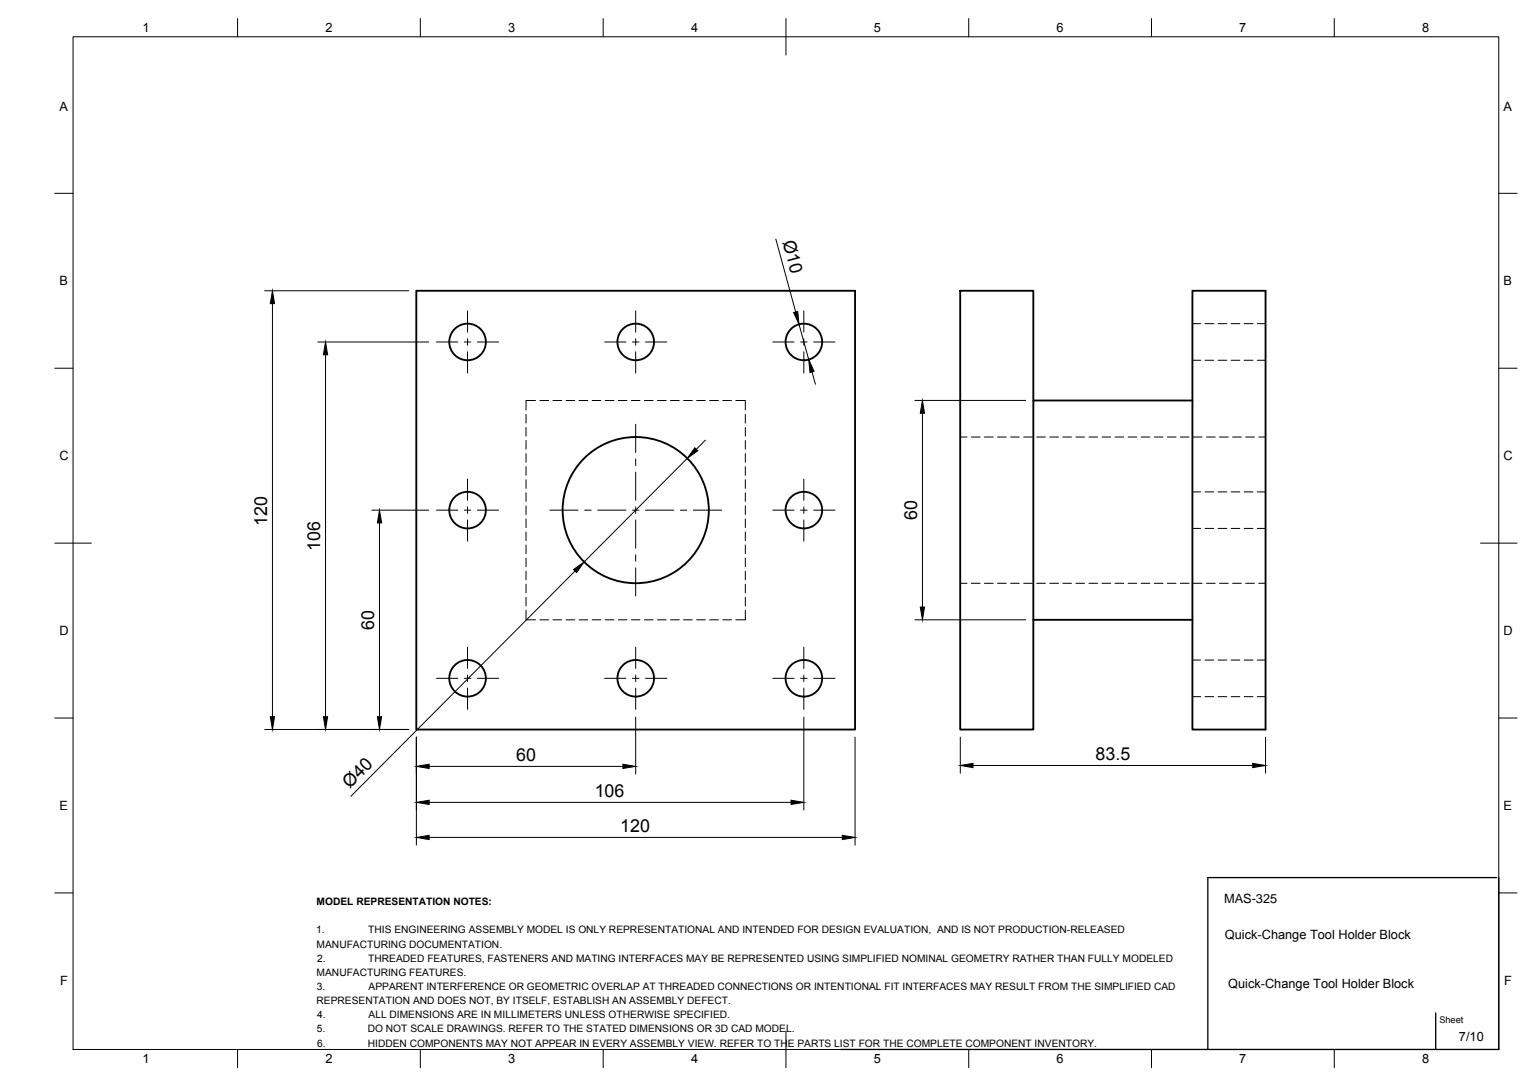
ISO-10303-21;
HEADER;
FILE_DESCRIPTION (('STEP AP214'),
    '1' );
FILE_NAME ('Quick-Change Tool Holder Block.step',
    '2026-10-08T01:23:29',
    ( '' ),
    ( '' ),
    'SwSTEP 2.0',
    'SolidWorks 2025',
    '' );
FILE_SCHEMA (( 'AUTOMOTIVE_DESIGN' ));
ENDSEC;

DATA;
#8=DIRECTION ( 'NONE',  ( 0.000000000000000000, 0.000000000000000000, -1.000000000000000000 ) ) ;
#231=DIRECTION ( 'NONE',  ( -0.000000000000000000, 1.000000000000000000, -0.000000000000000000 ) ) ;
#235=AXIS2_PLACEMENT_3D ( 'NONE', #29797, #45849, #41895 ) ;
#469=EDGE_LOOP ( 'NONE', ( #38599, #878, #20633, #16037 ) ) ;
#500=AXIS2_PLACEMENT_3D ( 'NONE', #889, #41099, #37682 ) ;
#509=DIRECTION ( 'NONE',  ( 0.000000000000000000, 1.000000000000000000, 0.000000000000000000 ) ) ;
#511=DIRECTION ( 'NONE',  ( 1.000000000000000000, -0.000000000000000000, 0.000000000000000000 ) ) ;
#519=CIRCLE ( 'NONE', #6403, 4.999999999999997335 ) ;
#529=( GEOMETRIC_REPRESENTATION_CONTEXT ( 3 ) GLOBAL_UNCERTAINTY_ASSIGNED_CONTEXT ( ( #31631 ) ) GLOBAL_UNIT_ASSIGNED_CONTEXT ( ( #33419, #33134, #45500 ) ) REPRESENTATION_CONTEXT ( 'NONE', 'WORKASPACE' ) );
#610=ADVANCED_FACE ( 'NONE', ( #10402 ), #26946, .F. ) ;
#630=ORIENTED_EDGE ( 'NONE', *, *, #47620, .F. ) ;
#643=ORIENTED_EDGE ( 'NONE', *, *, #44701, .T. ) ;
#683=EDGE_LOOP ( 'NONE', ( #15147, #11656, #13583, #27814 ) ) ;
#690=FACE_OUTER_BOUND ( 'NONE', #23025, .T. ) ;
#746=CARTESIAN_POINT ( 'NONE',  ( -46.00000000000000711, 0.000000000000000000, 8.673617379884035472E-15 ) ) ;
#755=VERTEX_POINT ( 'NONE', #51930 ) ;
#805=CARTESIAN_POINT ( 'NONE',  ( 46.00000000000000711, 0.000000000000000000, 41.00000000000000000 ) ) ;
#835=DIRECTION ( 'NONE',  ( 0.000000000000000000, 1.000000000000000000, 0.000000000000000000 ) ) ;
#848=ORIENTED_EDGE ( 'NONE', *, *, #2477, .T. ) ;
#878=ORIENTED_EDGE ( 'NONE', *, *, #33812, .F. ) ;
#889=CARTESIAN_POINT ( 'NONE',  ( 46.00000000000000711, 20.00000000000000000, 46.00000000000000000 ) ) ;
#902=EDGE_CURVE ( 'NONE', #32022, #7418, #51728, .T. ) ;
#905=DIRECTION ( 'NONE',  ( 0.000000000000000000, 0.000000000000000000, 1.000000000000000000 ) ) ;
#956=DIRECTION ( 'NONE',  ( 0.000000000000000000, 0.000000000000000000, -1.000000000000000000 ) ) ;
#984=CARTESIAN_POINT ( 'NONE',  ( -46.00000000000000711, 20.00000000000000000, 51.00000000000000000 ) ) ;
#1030=CIRCLE ( 'NONE', #8567, 4.999999999999997335 ) ;
#1039=EDGE_LOOP ( 'NONE', ( #32156, #50027, #34356, #41255 ) ) ;
#1073=SURFACE_SIDE_STYLE ('',( #5041 ) ) ;
#1080=PLANE ( 'NONE',  #27310 ) ;
#1090=DIRECTION ( 'NONE',  ( 0.000000000000000000, 0.000000000000000000, 1.000000000000000000 ) ) ;
#1094=DIRECTION ( 'NONE',  ( 0.000000000000000000, 0.000000000000000000, 1.000000000000000000 ) ) ;
#1126=VERTEX_POINT ( 'NONE', #22089 ) ;
#1141=MANIFOLD_SOLID_BREP ( 'Cut-Extrude1', #17058 ) ;
#1185=EDGE_LOOP ( 'NONE', ( #30507, #5255 ) ) ;
#1316=LINE ( 'NONE', #8951, #2361 ) ;
#1322=ORIENTED_EDGE ( 'NONE', *, *, #37609, .F. ) ;
#1346=CARTESIAN_POINT ( 'NONE',  ( -60.00000000000000000, 20.00000000000000000, 60.00000000000000711 ) ) ;
#1349=VERTEX_POINT ( 'NONE', #40428 ) ;
#1372=STYLED_ITEM ( 'NONE', ( #29978 ), #1141 ) ;
#1532=DIRECTION ( 'NONE',  ( 0.000000000000000000, -1.000000000000000000, 0.000000000000000000 ) ) ;
#1533=DIRECTION ( 'NONE',  ( 0.000000000000000000, 0.000000000000000000, -1.000000000000000000 ) ) ;
#1580=CARTESIAN_POINT ( 'NONE',  ( -60.00000000000000000, 0.000000000000000000, 60.00000000000000711 ) ) ;
#1620=DIRECTION ( 'NONE',  ( 1.000000000000000000, -0.000000000000000000, 0.000000000000000000 ) ) ;
#1628=LINE ( 'NONE', #13193, #27463 ) ;
#1634=ORIENTED_EDGE ( 'NONE', *, *, #11718, .F. ) ;
#1637=EDGE_CURVE ( 'NONE', #4347, #48702, #44495, .T. ) ;
#1686=ORIENTED_EDGE ( 'NONE', *, *, #8609, .T. ) ;
#1690=FACE_OUTER_BOUND ( 'NONE', #43640, .T. ) ;
#1791=DIRECTION ( 'NONE',  ( 0.000000000000000000, 0.000000000000000000, 1.000000000000000000 ) ) ;
#1796=DIRECTION ( 'NONE',  ( 0.000000000000000000, 0.000000000000000000, -1.000000000000000000 ) ) ;
#1921=EDGE_CURVE ( 'NONE', #24400, #35572, #31639, .T. ) ;
#1968=CARTESIAN_POINT ( 'NONE',  ( 46.00000000000000000, 20.00000000000000000, -4.999999999999997335 ) ) ;
#2088=VERTEX_POINT ( 'NONE', #36530 ) ;
#2096=DIRECTION ( 'NONE',  ( 0.000000000000000000, -1.000000000000000000, 0.000000000000000000 ) ) ;
#2101=VERTEX_POINT ( 'NONE', #805 ) ;
#2131=DIRECTION ( 'NONE',  ( 0.000000000000000000, 1.000000000000000000, 0.000000000000000000 ) ) ;
#2170=DIRECTION ( 'NONE',  ( 1.000000000000000000, -0.000000000000000000, 0.000000000000000000 ) ) ;
#2214=DIRECTION ( 'NONE',  ( 0.000000000000000000, 1.000000000000000000, 0.000000000000000000 ) ) ;
#2313=AXIS2_PLACEMENT_3D ( 'NONE', #18632, #34644, #50691 ) ;
#2361=VECTOR ( 'NONE', #24717, 1000.000000000000000 ) ;
#2426=CARTESIAN_POINT ( 'NONE',  ( 46.00000000000000000, 20.00000000000000000, 0.000000000000000000 ) ) ;
#2477=EDGE_CURVE ( 'NONE', #17289, #7125, #26422, .T. ) ;
#2494=CIRCLE ( 'NONE', #9212, 4.999999999999997335 ) ;
#2589=CARTESIAN_POINT ( 'NONE',  ( 0.000000000000000000, 0.000000000000000000, 0.000000000000000000 ) ) ;
#2614=ORIENTED_EDGE ( 'NONE', *, *, #31482, .F. ) ;
#2675=VECTOR ( 'NONE', #3987, 1000.000000000000000 ) ;
#2678=CARTESIAN_POINT ( 'NONE',  ( -46.00000000000000711, 0.000000000000000000, 51.00000000000000000 ) ) ;
#2740=UNCERTAINTY_MEASURE_WITH_UNIT (LENGTH_MEASURE( 1.000000000000000082E-05 ), #29982, 'distance_accuracy_value', 'NONE');
#2781=FACE_BOUND ( 'NONE', #44782, .T. ) ;
#2946=AXIS2_PLACEMENT_3D ( 'NONE', #746, #12029, #48846 ) ;
#2982=EDGE_LOOP ( 'NONE', ( #34516, #40352, #15843, #39033 ) ) ;
#2988=VECTOR ( 'NONE', #2170, 1000.000000000000000 ) ;
#3042=FACE_BOUND ( 'NONE', #22300, .T. ) ;
#3127=ORIENTED_EDGE ( 'NONE', *, *, #18949, .T. ) ;
#3185=FACE_OUTER_BOUND ( 'NONE', #37672, .T. ) ;
#3397=DIRECTION ( 'NONE',  ( 0.000000000000000000, 1.000000000000000000, 0.000000000000000000 ) ) ;
#3409=EDGE_CURVE ( 'NONE', #44223, #31469, #13220, .T. ) ;
#3423=DIRECTION ( 'NONE',  ( 0.000000000000000000, 0.000000000000000000, 1.000000000000000000 ) ) ;
#3531=CARTESIAN_POINT ( 'NONE',  ( 3.686287386450715076E-15, 20.00000000000000000, -51.00000000000000711 ) ) ;
#3541=CARTESIAN_POINT ( 'NONE',  ( -46.00000000000000711, 20.00000000000000000, 46.00000000000000000 ) ) ;
#3568=ORIENTED_EDGE ( 'NONE', *, *, #4402, .F. ) ;
#3630=CARTESIAN_POINT ( 'NONE',  ( 60.00000000000001421, -43.50000000000000000, 0.000000000000000000 ) ) ;
#3641=ORIENTED_EDGE ( 'NONE', *, *, #27551, .T. ) ;
#3670=DIRECTION ( 'NONE',  ( -0.000000000000000000, -1.000000000000000000, -0.000000000000000000 ) ) ;
#3714=CARTESIAN_POINT ( 'NONE',  ( 0.000000000000000000, 0.000000000000000000, 0.000000000000000000 ) ) ;
#3813=AXIS2_PLACEMENT_3D ( 'NONE', #22588, #41779, #50196 ) ;
#3855=DIRECTION ( 'NONE',  ( 0.000000000000000000, 0.000000000000000000, -1.000000000000000000 ) ) ;
#3861=ORIENTED_EDGE ( 'NONE', *, *, #27551, .F. ) ;
#3882=VECTOR ( 'NONE', #3670, 1000.000000000000000 ) ;
#3883=CYLINDRICAL_SURFACE ( 'NONE', #28633, 4.999999999999997335 ) ;
#3895=VECTOR ( 'NONE', #11796, 1000.000000000000000 ) ;
#3902=ORIENTED_EDGE ( 'NONE', *, *, #34227, .F. ) ;
#3904=LINE ( 'NONE', #3630, #38504 ) ;
#3936=CARTESIAN_POINT ( 'NONE',  ( 0.000000000000000000, -63.50000000000000000, 0.000000000000000000 ) ) ;
#3954=CIRCLE ( 'NONE', #45083, 4.999999999999997335 ) ;
#3985=CARTESIAN_POINT ( 'NONE',  ( -60.00000000000000000, 20.00000000000000000, -60.00000000000000711 ) ) ;
#3987=DIRECTION ( 'NONE',  ( -0.000000000000000000, -1.000000000000000000, -0.000000000000000000 ) ) ;
#4040=VECTOR ( 'NONE', #41244, 1000.000000000000000 ) ;
#4073=FACE_OUTER_BOUND ( 'NONE', #29955, .T. ) ;
#4079=ORIENTED_EDGE ( 'NONE', *, *, #24879, .T. ) ;
#4080=CARTESIAN_POINT ( 'NONE',  ( 46.00000000000000711, 0.000000000000000000, -41.00000000000000000 ) ) ;
#4147=EDGE_CURVE ( 'NONE', #15921, #22734, #9361, .T. ) ;
#4244=LINE ( 'NONE', #7662, #2675 ) ;
#4347=VERTEX_POINT ( 'NONE', #31648 ) ;
#4402=EDGE_CURVE ( 'NONE', #12957, #38011, #44515, .T. ) ;
#4405=DIRECTION ( 'NONE',  ( -0.000000000000000000, -1.000000000000000000, -0.000000000000000000 ) ) ;
#4414=EDGE_CURVE ( 'NONE', #28503, #18767, #48724, .T. ) ;
#4431=ORIENTED_EDGE ( 'NONE', *, *, #23553, .F. ) ;
#4572=CARTESIAN_POINT ( 'NONE',  ( 60.00000000000001421, 0.000000000000000000, 60.00000000000000711 ) ) ;
#4693=FACE_BOUND ( 'NONE', #20510, .T. ) ;
#4770=ORIENTED_EDGE ( 'NONE', *, *, #41010, .T. ) ;
#4804=ORIENTED_EDGE ( 'NONE', *, *, #25842, .T. ) ;
#4819=EDGE_CURVE ( 'NONE', #1349, #12957, #519, .T. ) ;
#4931=EDGE_LOOP ( 'NONE', ( #26759, #38319, #25353, #4431 ) ) ;
#4984=PRODUCT_CONTEXT ( 'NONE', #41108, 'mechanical' ) ;
#5041=SURFACE_STYLE_FILL_AREA ( #49956 ) ;
#5146=VERTEX_POINT ( 'NONE', #20149 ) ;
#5255=ORIENTED_EDGE ( 'NONE', *, *, #7025, .T. ) ;
#5265=CARTESIAN_POINT ( 'NONE',  ( 3.686287386450715076E-15, 0.000000000000000000, -51.00000000000000711 ) ) ;
#5492=VERTEX_POINT ( 'NONE', #38955 ) ;
#5593=ORIENTED_EDGE ( 'NONE', *, *, #21466, .F. ) ;
#5636=DIRECTION ( 'NONE',  ( 0.000000000000000000, 0.000000000000000000, -1.000000000000000000 ) ) ;
#5643=CIRCLE ( 'NONE', #22389, 4.999999999999997335 ) ;
#5650=CYLINDRICAL_SURFACE ( 'NONE', #44597, 4.999999999999997335 ) ;
#5685=CARTESIAN_POINT ( 'NONE',  ( 46.00000000000000711, 20.00000000000000000, -41.00000000000000000 ) ) ;
#5691=EDGE_LOOP ( 'NONE', ( #30462, #46109 ) ) ;
#5693=ORIENTED_EDGE ( 'NONE', *, *, #44701, .F. ) ;
#5706=DIRECTION ( 'NONE',  ( 0.000000000000000000, 0.000000000000000000, -1.000000000000000000 ) ) ;
#5754=EDGE_CURVE ( 'NONE', #12927, #38011, #3954, .T. ) ;
#5761=CARTESIAN_POINT ( 'NONE',  ( 46.00000000000000711, 0.000000000000000000, 46.00000000000000000 ) ) ;
#5767=DIRECTION ( 'NONE',  ( 0.000000000000000000, 1.000000000000000000, 0.000000000000000000 ) ) ;
#5781=VECTOR ( 'NONE', #38082, 1000.000000000000000 ) ;
#5784=FACE_BOUND ( 'NONE', #7278, .T. ) ;
#5789=EDGE_CURVE ( 'NONE', #7450, #24959, #1628, .T. ) ;
#5792=DIRECTION ( 'NONE',  ( 0.000000000000000000, 0.000000000000000000, 1.000000000000000000 ) ) ;
#5818=CARTESIAN_POINT ( 'NONE',  ( 46.00000000000000000, 0.000000000000000000, 4.999999999999997335 ) ) ;
#5827=CARTESIAN_POINT ( 'NONE',  ( -60.00000000000000000, 20.00000000000000000, 60.00000000000000711 ) ) ;
#5888=PRODUCT ( 'Quick-Change Tool Holder Block', 'Quick-Change Tool Holder Block', '', ( #4984 ) ) ;
#5895=ORIENTED_EDGE ( 'NONE', *, *, #17945, .T. ) ;
#5901=AXIS2_PLACEMENT_3D ( 'NONE', #21940, #30584, #50842 ) ;
#6015=DIRECTION ( 'NONE',  ( 0.000000000000000000, -1.000000000000000000, 0.000000000000000000 ) ) ;
#6058=CARTESIAN_POINT ( 'NONE',  ( 0.000000000000000000, -43.50000000000000000, 60.00000000000000711 ) ) ;
#6066=CARTESIAN_POINT ( 'NONE',  ( -46.00000000000000711, 20.00000000000000000, 51.00000000000000000 ) ) ;
#6079=AXIS2_PLACEMENT_3D ( 'NONE', #11818, #39421, #3423 ) ;
#6101=EDGE_CURVE ( 'NONE', #39324, #2101, #27838, .T. ) ;
#6133=CARTESIAN_POINT ( 'NONE',  ( 0.000000000000000000, -63.50000000000000000, 60.00000000000000711 ) ) ;
#6145=VERTEX_POINT ( 'NONE', #39918 ) ;
#6217=CARTESIAN_POINT ( 'NONE',  ( 60.00000000000001421, 20.00000000000000000, 60.00000000000000711 ) ) ;
#6247=ORIENTED_EDGE ( 'NONE', *, *, #1637, .T. ) ;
#6348=AXIS2_PLACEMENT_3D ( 'NONE', #34789, #46647, #41718 ) ;
#6392=CARTESIAN_POINT ( 'NONE',  ( -46.00000000000000711, 20.00000000000000000, 41.00000000000000000 ) ) ;
#6403=AXIS2_PLACEMENT_3D ( 'NONE', #26477, #37548, #1791 ) ;
#6461=AXIS2_PLACEMENT_3D ( 'NONE', #41940, #49327, #37993 ) ;
#6502=ORIENTED_EDGE ( 'NONE', *, *, #34896, .F. ) ;
#6529=DIRECTION ( 'NONE',  ( 0.000000000000000000, 1.000000000000000000, -0.000000000000000000 ) ) ;
#6548=ORIENTED_EDGE ( 'NONE', *, *, #40003, .F. ) ;
#6553=CARTESIAN_POINT ( 'NONE',  ( -46.00000000000000711, 0.000000000000000000, 46.00000000000000000 ) ) ;
#6561=FACE_OUTER_BOUND ( 'NONE', #21554, .T. ) ;
#6707=ORIENTED_EDGE ( 'NONE', *, *, #7167, .T. ) ;
#6734=EDGE_CURVE ( 'NONE', #5146, #10970, #33743, .T. ) ;
#6854=EDGE_CURVE ( 'NONE', #51787, #22734, #42666, .T. ) ;
#7025=EDGE_CURVE ( 'NONE', #7418, #32022, #49672, .T. ) ;
#7068=CARTESIAN_POINT ( 'NONE',  ( 46.00000000000000711, 0.000000000000000000, -46.00000000000000000 ) ) ;
#7093=CARTESIAN_POINT ( 'NONE',  ( 3.686287386450715076E-15, 20.00000000000000000, -46.00000000000000711 ) ) ;
#7111=VECTOR ( 'NONE', #5767, 1000.000000000000000 ) ;
#7125=VERTEX_POINT ( 'NONE', #46052 ) ;
#7126=EDGE_LOOP ( 'NONE', ( #30101, #33075, #43603, #25151 ) ) ;
#7149=ORIENTED_EDGE ( 'NONE', *, *, #48869, .T. ) ;
#7161=CIRCLE ( 'NONE', #27287, 4.999999999999997335 ) ;
#7167=EDGE_CURVE ( 'NONE', #32303, #51023, #36261, .T. ) ;
#7209=CARTESIAN_POINT ( 'NONE',  ( 60.00000000000001421, -63.50000000000000000, 60.00000000000000711 ) ) ;
#7264=DIRECTION ( 'NONE',  ( -0.000000000000000000, -1.000000000000000000, -0.000000000000000000 ) ) ;
#7278=EDGE_LOOP ( 'NONE', ( #48814, #44338 ) ) ;
#7334=ADVANCED_FACE ( 'NONE', ( #32309 ), #40203, .F. ) ;
#7418=VERTEX_POINT ( 'NONE', #37037 ) ;
#7450=VERTEX_POINT ( 'NONE', #13913 ) ;
#7488=VECTOR ( 'NONE', #38142, 1000.000000000000000 ) ;
#7497=CYLINDRICAL_SURFACE ( 'NONE', #35759, 4.999999999999997335 ) ;
#7503=LINE ( 'NONE', #8008, #28662 ) ;
#7516=FACE_BOUND ( 'NONE', #18343, .T. ) ;
#7524=ORIENTED_EDGE ( 'NONE', *, *, #44163, .F. ) ;
#7547=ORIENTED_EDGE ( 'NONE', *, *, #36563, .F. ) ;
#7557=ORIENTED_EDGE ( 'NONE', *, *, #37236, .T. ) ;
#7662=CARTESIAN_POINT ( 'NONE',  ( 46.00000000000000000, 20.00000000000000000, 4.999999999999997335 ) ) ;
#7765=PLANE ( 'NONE',  #14213 ) ;
#8008=CARTESIAN_POINT ( 'NONE',  ( 0.000000000000000000, -43.50000000000000000, 30.00000000000000355 ) ) ;
#8064=DIRECTION ( 'NONE',  ( 0.000000000000000000, 0.000000000000000000, -1.000000000000000000 ) ) ;
#8088=MECHANICAL_DESIGN_GEOMETRIC_PRESENTATION_REPRESENTATION('',(#1372),#529);
#8215=CARTESIAN_POINT ( 'NONE',  ( -60.00000000000000000, -63.50000000000000000, 60.00000000000000711 ) ) ;
#8284=AXIS2_PLACEMENT_3D ( 'NONE', #30164, #30408, #1533 ) ;
#8332=CYLINDRICAL_SURFACE ( 'NONE', #28030, 4.999999999999997335 ) ;
#8342=AXIS2_PLACEMENT_3D ( 'NONE', #33031, #17022, #40378 ) ;
#8393=CARTESIAN_POINT ( 'NONE',  ( -60.00000000000000000, 20.00000000000000000, 60.00000000000000711 ) ) ;
#8412=EDGE_LOOP ( 'NONE', ( #41893, #848 ) ) ;
#8438=DIRECTION ( 'NONE',  ( 1.000000000000000000, 0.000000000000000000, 0.000000000000000000 ) ) ;
#8551=EDGE_CURVE ( 'NONE', #23514, #28503, #43677, .T. ) ;
#8567=AXIS2_PLACEMENT_3D ( 'NONE', #48358, #509, #40450 ) ;
#8609=EDGE_CURVE ( 'NONE', #2088, #36416, #37552, .T. ) ;
#8665=CARTESIAN_POINT ( 'NONE',  ( 1.734723475976807094E-15, 20.00000000000000000, 41.00000000000000711 ) ) ;
#8716=FACE_BOUND ( 'NONE', #1185, .T. ) ;
#8752=PRODUCT_DEFINITION ( 'UNKNOWN', '', #25890, #46912 ) ;
#8951=CARTESIAN_POINT ( 'NONE',  ( -30.00000000000000000, -43.50000000000000000, 30.00000000000000355 ) ) ;
#8988=PLANE ( 'NONE',  #17210 ) ;
#9019=AXIS2_PLACEMENT_3D ( 'NONE', #30402, #43540, #46452 ) ;
#9124=EDGE_CURVE ( 'NONE', #35572, #24400, #23996, .T. ) ;
#9162=CARTESIAN_POINT ( 'NONE',  ( -46.00000000000000711, 20.00000000000000000, -46.00000000000000000 ) ) ;
#9166=DIRECTION ( 'NONE',  ( 0.000000000000000000, 0.000000000000000000, -1.000000000000000000 ) ) ;
#9212=AXIS2_PLACEMENT_3D ( 'NONE', #2426, #30523, #22394 ) ;
#9268=EDGE_LOOP ( 'NONE', ( #38964, #27022 ) ) ;
#9361=LINE ( 'NONE', #41927, #24178 ) ;
#9407=CIRCLE ( 'NONE', #36251, 4.999999999999997335 ) ;
#9439=CARTESIAN_POINT ( 'NONE',  ( 4.298610786024391605E-15, 20.00000000000000000, -41.00000000000000711 ) ) ;
#9671=AXIS2_PLACEMENT_3D ( 'NONE', #40075, #48759, #36662 ) ;
#9712=VECTOR ( 'NONE', #27639, 1000.000000000000000 ) ;
#9733=ORIENTED_EDGE ( 'NONE', *, *, #7167, .F. ) ;
#9982=DIRECTION ( 'NONE',  ( 0.000000000000000000, 1.000000000000000000, 0.000000000000000000 ) ) ;
#10076=ORIENTED_EDGE ( 'NONE', *, *, #21894, .T. ) ;
#10114=CARTESIAN_POINT ( 'NONE',  ( 30.00000000000000711, 0.000000000000000000, -30.00000000000000355 ) ) ;
#10243=AXIS2_PLACEMENT_3D ( 'NONE', #46644, #46908, #22717 ) ;
#10276=LINE ( 'NONE', #34446, #28627 ) ;
#10402=FACE_OUTER_BOUND ( 'NONE', #33728, .T. ) ;
#10425=ADVANCED_FACE ( 'NONE', ( #48600 ), #24662, .F. ) ;
#10445=DIRECTION ( 'NONE',  ( 0.000000000000000000, 0.000000000000000000, -1.000000000000000000 ) ) ;
#10511=AXIS2_PLACEMENT_3D ( 'NONE', #9162, #44633, #25189 ) ;
#10565=DIRECTION ( 'NONE',  ( -0.000000000000000000, -1.000000000000000000, -0.000000000000000000 ) ) ;
#10748=CARTESIAN_POINT ( 'NONE',  ( -60.00000000000000000, 20.00000000000000000, 60.00000000000000711 ) ) ;
#10832=EDGE_CURVE ( 'NONE', #6145, #23787, #1316, .T. ) ;
#10852=CIRCLE ( 'NONE', #8342, 4.999999999999997335 ) ;
#10928=DIRECTION ( 'NONE',  ( 0.000000000000000000, 0.000000000000000000, 1.000000000000000000 ) ) ;
#10970=VERTEX_POINT ( 'NONE', #47805 ) ;
#11051=VECTOR ( 'NONE', #33995, 1000.000000000000000 ) ;
#11070=CARTESIAN_POINT ( 'NONE',  ( 2.347046875550483230E-15, 20.00000000000000000, 51.00000000000000711 ) ) ;
#11100=CARTESIAN_POINT ( 'NONE',  ( -60.00000000000000000, 0.000000000000000000, 60.00000000000000711 ) ) ;
#11107=PLANE ( 'NONE',  #19321 ) ;
#11209=CARTESIAN_POINT ( 'NONE',  ( -46.00000000000000711, 0.000000000000000000, 41.00000000000000000 ) ) ;
#11223=EDGE_CURVE ( 'NONE', #33816, #30271, #34168, .T. ) ;
#11297=DIRECTION ( 'NONE',  ( -0.000000000000000000, -1.000000000000000000, -0.000000000000000000 ) ) ;
#11322=CIRCLE ( 'NONE', #10511, 4.999999999999997335 ) ;
#11435=DIRECTION ( 'NONE',  ( 0.000000000000000000, -1.000000000000000000, 0.000000000000000000 ) ) ;
#11513=CARTESIAN_POINT ( 'NONE',  ( 0.000000000000000000, 20.00000000000000355, 0.000000000000000000 ) ) ;
#11581=CARTESIAN_POINT ( 'NONE',  ( 1.734723475976807094E-15, 20.00000000000000000, 46.00000000000000711 ) ) ;
#11638=EDGE_LOOP ( 'NONE', ( #27597, #630 ) ) ;
#11656=ORIENTED_EDGE ( 'NONE', *, *, #4819, .T. ) ;
#11667=ORIENTED_EDGE ( 'NONE', *, *, #24509, .F. ) ;
#11671=CIRCLE ( 'NONE', #49477, 4.999999999999997335 ) ;
#11718=EDGE_CURVE ( 'NONE', #23787, #39696, #18349, .T. ) ;
#11729=CARTESIAN_POINT ( 'NONE',  ( -46.00000000000000711, 20.00000000000000000, 46.00000000000000000 ) ) ;
#11742=CARTESIAN_POINT ( 'NONE',  ( 46.00000000000000711, 20.00000000000000000, 46.00000000000000000 ) ) ;
#11748=ORIENTED_EDGE ( 'NONE', *, *, #41081, .T. ) ;
#11753=ADVANCED_FACE ( 'NONE', ( #18078 ), #14150, .F. ) ;
#11796=DIRECTION ( 'NONE',  ( 0.000000000000000000, 0.000000000000000000, -1.000000000000000000 ) ) ;
#11818=CARTESIAN_POINT ( 'NONE',  ( 46.00000000000000000, 0.000000000000000000, 0.000000000000000000 ) ) ;
#11911=AXIS2_PLACEMENT_3D ( 'NONE', #44476, #21073, #1094 ) ;
#11924=DIRECTION ( 'NONE',  ( -0.000000000000000000, -1.000000000000000000, -0.000000000000000000 ) ) ;
#11963=ORIENTED_EDGE ( 'NONE', *, *, #6101, .F. ) ;
#12029=DIRECTION ( 'NONE',  ( 0.000000000000000000, 1.000000000000000000, 0.000000000000000000 ) ) ;
#12149=VECTOR ( 'NONE', #44728, 1000.000000000000000 ) ;
#12271=ORIENTED_EDGE ( 'NONE', *, *, #23194, .F. ) ;
#12645=EDGE_LOOP ( 'NONE', ( #5693, #46324, #10076, #30400 ) ) ;
#12839=LINE ( 'NONE', #36483, #3895 ) ;
#12895=ORIENTED_EDGE ( 'NONE', *, *, #3409, .T. ) ;
#12927=VERTEX_POINT ( 'NONE', #51946 ) ;
#12930=DIRECTION ( 'NONE',  ( -0.000000000000000000, 0.000000000000000000, 1.000000000000000000 ) ) ;
#12957=VERTEX_POINT ( 'NONE', #27489 ) ;
#12959=CIRCLE ( 'NONE', #42338, 4.999999999999997335 ) ;
#13006=DIRECTION ( 'NONE',  ( -0.000000000000000000, -1.000000000000000000, -0.000000000000000000 ) ) ;
#13137=ADVANCED_FACE ( 'NONE', ( #34023 ), #50069, .F. ) ;
#13193=CARTESIAN_POINT ( 'NONE',  ( 60.00000000000001421, 20.00000000000000000, -60.00000000000000711 ) ) ;
#13220=CIRCLE ( 'NONE', #21630, 20.00000000000000000 ) ;
#13239=VECTOR ( 'NONE', #41923, 1000.000000000000000 ) ;
#13246=ORIENTED_EDGE ( 'NONE', *, *, #14564, .F. ) ;
#13548=LINE ( 'NONE', #5685, #13239 ) ;
#13583=ORIENTED_EDGE ( 'NONE', *, *, #4402, .T. ) ;
#13636=ORIENTED_EDGE ( 'NONE', *, *, #21463, .T. ) ;
#13675=VECTOR ( 'NONE', #8064, 1000.000000000000000 ) ;
#13686=DIRECTION ( 'NONE',  ( 0.000000000000000000, 0.000000000000000000, -1.000000000000000000 ) ) ;
#13707=DIRECTION ( 'NONE',  ( 0.000000000000000000, 0.000000000000000000, 1.000000000000000000 ) ) ;
#13780=CYLINDRICAL_SURFACE ( 'NONE', #235, 20.00000000000000000 ) ;
#13795=AXIS2_PLACEMENT_3D ( 'NONE', #19327, #22745, #39289 ) ;
#13896=VERTEX_POINT ( 'NONE', #34153 ) ;
#13913=CARTESIAN_POINT ( 'NONE',  ( 60.00000000000001421, 20.00000000000000000, -60.00000000000000711 ) ) ;
#13953=SURFACE_STYLE_USAGE ( .BOTH. , #1073 ) ;
#14016=DIRECTION ( 'NONE',  ( -0.000000000000000000, -1.000000000000000000, -0.000000000000000000 ) ) ;
#14051=CIRCLE ( 'NONE', #9019, 4.999999999999997335 ) ;
#14080=CARTESIAN_POINT ( 'NONE',  ( -46.00000000000000711, 20.00000000000000000, -51.00000000000000000 ) ) ;
#14150=CYLINDRICAL_SURFACE ( 'NONE', #8284, 4.999999999999997335 ) ;
#14164=EDGE_CURVE ( 'NONE', #7125, #17289, #7161, .T. ) ;
#14177=DIRECTION ( 'NONE',  ( 0.000000000000000000, 0.000000000000000000, -1.000000000000000000 ) ) ;
#14213=AXIS2_PLACEMENT_3D ( 'NONE', #47208, #11435, #50891 ) ;
#14235=CARTESIAN_POINT ( 'NONE',  ( 46.00000000000000000, 20.00000000000000000, 0.000000000000000000 ) ) ;
#14287=DIRECTION ( 'NONE',  ( 1.000000000000000000, -0.000000000000000000, 0.000000000000000000 ) ) ;
#14299=DIRECTION ( 'NONE',  ( -0.000000000000000000, 0.000000000000000000, 1.000000000000000000 ) ) ;
#14438=ORIENTED_EDGE ( 'NONE', *, *, #27691, .T. ) ;
#14440=CYLINDRICAL_SURFACE ( 'NONE', #3813, 4.999999999999997335 ) ;
#14442=EDGE_CURVE ( 'NONE', #31192, #41489, #26471, .T. ) ;
#14456=EDGE_LOOP ( 'NONE', ( #27565, #34564 ) ) ;
#14458=VECTOR ( 'NONE', #13006, 1000.000000000000000 ) ;
#14462=VERTEX_POINT ( 'NONE', #7209 ) ;
#14531=VECTOR ( 'NONE', #15083, 1000.000000000000000 ) ;
#14554=EDGE_LOOP ( 'NONE', ( #19755, #1634, #48038, #40314 ) ) ;
#14564=EDGE_CURVE ( 'NONE', #36416, #31403, #19547, .T. ) ;
#14581=EDGE_CURVE ( 'NONE', #22734, #23787, #19307, .T. ) ;
#14674=DIRECTION ( 'NONE',  ( 0.000000000000000000, 0.000000000000000000, -1.000000000000000000 ) ) ;
#14767=VERTEX_POINT ( 'NONE', #2678 ) ;
#14799=ORIENTED_EDGE ( 'NONE', *, *, #6101, .T. ) ;
#14803=CYLINDRICAL_SURFACE ( 'NONE', #50951, 4.999999999999997335 ) ;
#14866=VECTOR ( 'NONE', #27897, 1000.000000000000000 ) ;
#15068=ORIENTED_EDGE ( 'NONE', *, *, #36892, .T. ) ;
#15078=DIRECTION ( 'NONE',  ( -0.000000000000000000, -0.000000000000000000, 1.000000000000000000 ) ) ;
#15083=DIRECTION ( 'NONE',  ( 1.000000000000000000, 0.000000000000000000, 5.782411586589357392E-17 ) ) ;
#15147=ORIENTED_EDGE ( 'NONE', *, *, #20275, .F. ) ;
#15195=AXIS2_PLACEMENT_3D ( 'NONE', #2589, #26228, #38325 ) ;
#15239=CIRCLE ( 'NONE', #26106, 4.999999999999997335 ) ;
#15277=CARTESIAN_POINT ( 'NONE',  ( 46.00000000000000711, 0.000000000000000000, 46.00000000000000000 ) ) ;
#15310=DIRECTION ( 'NONE',  ( 0.000000000000000000, 0.000000000000000000, -1.000000000000000000 ) ) ;
#15330=DIRECTION ( 'NONE',  ( 0.000000000000000000, 1.000000000000000000, 0.000000000000000000 ) ) ;
#15332=CIRCLE ( 'NONE', #16161, 4.999999999999997335 ) ;
#15420=DIRECTION ( 'NONE',  ( 0.000000000000000000, 0.000000000000000000, -1.000000000000000000 ) ) ;
#15504=ADVANCED_BREP_SHAPE_REPRESENTATION ( '', ( #1141, #31742 ), #35946 ) ;
#15505=CYLINDRICAL_SURFACE ( 'NONE', #20527, 20.00000000000000000 ) ;
#15530=CYLINDRICAL_SURFACE ( 'NONE', #22671, 4.999999999999997335 ) ;
#15639=SHAPE_REPRESENTATION ( 'Quick-Change Tool Holder Block', ( #31742 ), #35946 ) ;
#15657=ORIENTED_EDGE ( 'NONE', *, *, #30163, .F. ) ;
#15695=CARTESIAN_POINT ( 'NONE',  ( -46.00000000000000711, 20.00000000000000000, -41.00000000000000000 ) ) ;
#15843=ORIENTED_EDGE ( 'NONE', *, *, #8609, .F. ) ;
#15921=VERTEX_POINT ( 'NONE', #10114 ) ;
#15986=EDGE_CURVE ( 'NONE', #47167, #13896, #12959, .T. ) ;
#16037=ORIENTED_EDGE ( 'NONE', *, *, #19576, .T. ) ;
#16161=AXIS2_PLACEMENT_3D ( 'NONE', #19453, #35474, #8 ) ;
#16211=FACE_OUTER_BOUND ( 'NONE', #34744, .T. ) ;
#16240=CARTESIAN_POINT ( 'NONE',  ( -60.00000000000000000, 20.00000000000000000, 60.00000000000000711 ) ) ;
#16248=DIRECTION ( 'NONE',  ( 0.000000000000000000, 0.000000000000000000, -1.000000000000000000 ) ) ;
#16254=ORIENTED_EDGE ( 'NONE', *, *, #43336, .F. ) ;
#16304=ORIENTED_EDGE ( 'NONE', *, *, #11223, .T. ) ;
#16421=DIRECTION ( 'NONE',  ( 0.000000000000000000, 0.000000000000000000, 1.000000000000000000 ) ) ;
#16439=LINE ( 'NONE', #31675, #50330 ) ;
#16515=LINE ( 'NONE', #29099, #49679 ) ;
#16551=FACE_OUTER_BOUND ( 'NONE', #24472, .T. ) ;
#16572=DIRECTION ( 'NONE',  ( 0.000000000000000000, 0.000000000000000000, -1.000000000000000000 ) ) ;
#16653=CARTESIAN_POINT ( 'NONE',  ( -30.00000000000000000, 0.000000000000000000, -30.00000000000000711 ) ) ;
#16655=AXIS2_PLACEMENT_3D ( 'NONE', #7068, #43320, #46498 ) ;
#16738=DIRECTION ( 'NONE',  ( -0.000000000000000000, -1.000000000000000000, -0.000000000000000000 ) ) ;
#16776=LINE ( 'NONE', #16240, #36959 ) ;
#16802=DIRECTION ( 'NONE',  ( -0.000000000000000000, -1.000000000000000000, -0.000000000000000000 ) ) ;
#16846=CARTESIAN_POINT ( 'NONE',  ( 60.00000000000001421, -43.50000000000000000, -60.00000000000000711 ) ) ;
#16862=PLANE ( 'NONE',  #23641 ) ;
#16878=CARTESIAN_POINT ( 'NONE',  ( -60.00000000000000000, 20.00000000000000000, -60.00000000000000711 ) ) ;
#16935=DIRECTION ( 'NONE',  ( 0.000000000000000000, 0.000000000000000000, -1.000000000000000000 ) ) ;
#17022=DIRECTION ( 'NONE',  ( 0.000000000000000000, 1.000000000000000000, 0.000000000000000000 ) ) ;
#17052=EDGE_LOOP ( 'NONE', ( #14438, #38483 ) ) ;
#17058=CLOSED_SHELL ( 'NONE', ( #31400, #24049, #29581, #25027, #51314, #40398, #26693, #31044, #13137, #24343, #26556, #610, #45273, #49490, #44587, #11753, #10425, #50405, #29293, #20482, #25479, #37895, #19524, #31142, #40186, #35954, #43324, #7334, #34253, #29817, #39417, #30173, #41188, #28477 ) ) ;
#17098=EDGE_CURVE ( 'NONE', #2088, #14462, #22986, .T. ) ;
#17155=DIRECTION ( 'NONE',  ( 1.000000000000000000, 0.000000000000000000, 0.000000000000000000 ) ) ;
#17172=EDGE_CURVE ( 'NONE', #5492, #25744, #48130, .T. ) ;
#17186=PRODUCT_DEFINITION_SHAPE ( 'NONE', 'NONE',  #8752 ) ;
#17210=AXIS2_PLACEMENT_3D ( 'NONE', #32881, #6015, #14177 ) ;
#17267=CYLINDRICAL_SURFACE ( 'NONE', #6461, 4.999999999999997335 ) ;
#17289=VERTEX_POINT ( 'NONE', #20011 ) ;
#17567=ORIENTED_EDGE ( 'NONE', *, *, #28137, .T. ) ;
#17605=EDGE_CURVE ( 'NONE', #12957, #1349, #44180, .T. ) ;
#17619=EDGE_LOOP ( 'NONE', ( #34868, #34787, #45073, #3902 ) ) ;
#17718=LINE ( 'NONE', #34249, #43222 ) ;
#17766=DIRECTION ( 'NONE',  ( -1.000000000000000000, -0.000000000000000000, -5.782411586589357392E-17 ) ) ;
#17805=ORIENTED_EDGE ( 'NONE', *, *, #24509, .T. ) ;
#17854=CARTESIAN_POINT ( 'NONE',  ( 1.734723475976807094E-15, 0.000000000000000000, 46.00000000000000711 ) ) ;
#17945=EDGE_CURVE ( 'NONE', #1126, #21250, #5643, .T. ) ;
#17984=CARTESIAN_POINT ( 'NONE',  ( 46.00000000000000711, 20.00000000000000000, -46.00000000000000000 ) ) ;
#18002=AXIS2_PLACEMENT_3D ( 'NONE', #47435, #35339, #16421 ) ;
#18045=LINE ( 'NONE', #42201, #47809 ) ;
#18078=FACE_OUTER_BOUND ( 'NONE', #683, .T. ) ;
#18094=CARTESIAN_POINT ( 'NONE',  ( -60.00000000000000000, -63.50000000000000000, -0.000000000000000000 ) ) ;
#18098=LINE ( 'NONE', #9439, #33263 ) ;
#18244=EDGE_LOOP ( 'NONE', ( #4804, #50055, #24012, #46903 ) ) ;
#18315=DIRECTION ( 'NONE',  ( -0.000000000000000000, -0.000000000000000000, 1.000000000000000000 ) ) ;
#18343=EDGE_LOOP ( 'NONE', ( #12895, #47356 ) ) ;
#18349=LINE ( 'NONE', #45685, #47762 ) ;
#18409=ORIENTED_EDGE ( 'NONE', *, *, #36563, .T. ) ;
#18588=VECTOR ( 'NONE', #5706, 1000.000000000000000 ) ;
#18632=CARTESIAN_POINT ( 'NONE',  ( -46.00000000000000711, 0.000000000000000000, -46.00000000000000000 ) ) ;
#18711=CARTESIAN_POINT ( 'NONE',  ( -46.00000000000000711, 20.00000000000000000, 46.00000000000000000 ) ) ;
#18767=VERTEX_POINT ( 'NONE', #31512 ) ;
#18949=EDGE_CURVE ( 'NONE', #39696, #15921, #12839, .T. ) ;
#19026=DIRECTION ( 'NONE',  ( 0.000000000000000000, 0.000000000000000000, 1.000000000000000000 ) ) ;
#19204=CARTESIAN_POINT ( 'NONE',  ( -46.00000000000000711, 0.000000000000000000, -41.00000000000000000 ) ) ;
#19212=DIRECTION ( 'NONE',  ( 0.000000000000000000, 0.000000000000000000, -1.000000000000000000 ) ) ;
#19220=DIRECTION ( 'NONE',  ( -0.000000000000000000, -1.000000000000000000, -0.000000000000000000 ) ) ;
#19307=LINE ( 'NONE', #39756, #50015 ) ;
#19309=ORIENTED_EDGE ( 'NONE', *, *, #23406, .F. ) ;
#19321=AXIS2_PLACEMENT_3D ( 'NONE', #50558, #14299, #38191 ) ;
#19327=CARTESIAN_POINT ( 'NONE',  ( 1.734723475976807094E-15, 20.00000000000000000, 46.00000000000000711 ) ) ;
#19349=ORIENTED_EDGE ( 'NONE', *, *, #43874, .F. ) ;
#19376=LINE ( 'NONE', #4572, #51630 ) ;
#19453=CARTESIAN_POINT ( 'NONE',  ( -46.00000000000000711, 0.000000000000000000, -46.00000000000000000 ) ) ;
#19504=LINE ( 'NONE', #31858, #34560 ) ;
#19521=ORIENTED_EDGE ( 'NONE', *, *, #20275, .T. ) ;
#19524=ADVANCED_FACE ( 'NONE', ( #31070 ), #14803, .F. ) ;
#19547=LINE ( 'NONE', #47931, #23957 ) ;
#19576=EDGE_CURVE ( 'NONE', #14462, #30271, #35271, .T. ) ;
#19698=DIRECTION ( 'NONE',  ( -0.000000000000000000, -1.000000000000000000, -0.000000000000000000 ) ) ;
#19710=ORIENTED_EDGE ( 'NONE', *, *, #51228, .F. ) ;
#19755=ORIENTED_EDGE ( 'NONE', *, *, #31482, .T. ) ;
#19827=DIRECTION ( 'NONE',  ( 0.000000000000000000, 1.000000000000000000, 0.000000000000000000 ) ) ;
#19854=CARTESIAN_POINT ( 'NONE',  ( 0.000000000000000000, -63.50000000000000000, -60.00000000000000711 ) ) ;
#19908=CARTESIAN_POINT ( 'NONE',  ( -46.00000000000000711, 20.00000000000000000, -46.00000000000000000 ) ) ;
#19932=CARTESIAN_POINT ( 'NONE',  ( -46.00000000000000711, 0.000000000000000000, 8.673617379884035472E-15 ) ) ;
#19958=DIRECTION ( 'NONE',  ( 0.000000000000000000, 0.000000000000000000, 1.000000000000000000 ) ) ;
#19959=ORIENTED_EDGE ( 'NONE', *, *, #21894, .F. ) ;
#19966=ORIENTED_EDGE ( 'NONE', *, *, #44128, .F. ) ;
#20011=CARTESIAN_POINT ( 'NONE',  ( -46.00000000000000711, 0.000000000000000000, 5.000000000000006217 ) ) ;
#20042=LINE ( 'NONE', #8215, #35833 ) ;
#20091=CARTESIAN_POINT ( 'NONE',  ( 46.00000000000000000, 20.00000000000000000, 0.000000000000000000 ) ) ;
#20149=CARTESIAN_POINT ( 'NONE',  ( 46.00000000000000711, 20.00000000000000000, 51.00000000000000000 ) ) ;
#20275=EDGE_CURVE ( 'NONE', #1349, #12927, #18098, .T. ) ;
#20281=LINE ( 'NONE', #51085, #44518 ) ;
#20400=LINE ( 'NONE', #24105, #13675 ) ;
#20453=PLANE ( 'NONE',  #37173 ) ;
#20482=ADVANCED_FACE ( 'NONE', ( #33548 ), #17267, .F. ) ;
#20510=EDGE_LOOP ( 'NONE', ( #7524, #38193, #27343, #29577 ) ) ;
#20527=AXIS2_PLACEMENT_3D ( 'NONE', #3936, #231, #19958 ) ;
#20633=ORIENTED_EDGE ( 'NONE', *, *, #17098, .T. ) ;
#20668=DIRECTION ( 'NONE',  ( -0.000000000000000000, -1.000000000000000000, -0.000000000000000000 ) ) ;
#20918=LINE ( 'NONE', #32978, #14458 ) ;
#20946=FACE_OUTER_BOUND ( 'NONE', #17619, .T. ) ;
#20958=ORIENTED_EDGE ( 'NONE', *, *, #36892, .F. ) ;
#21000=SHAPE_DEFINITION_REPRESENTATION ( #17186, #15639 ) ;
#21073=DIRECTION ( 'NONE',  ( 0.000000000000000000, 1.000000000000000000, 0.000000000000000000 ) ) ;
#21124=FACE_OUTER_BOUND ( 'NONE', #1039, .T. ) ;
#21132=DIRECTION ( 'NONE',  ( 0.000000000000000000, 0.000000000000000000, -1.000000000000000000 ) ) ;
#21185=CIRCLE ( 'NONE', #6079, 4.999999999999997335 ) ;
#21248=AXIS2_PLACEMENT_3D ( 'NONE', #6217, #38257, #10928 ) ;
#21250=VERTEX_POINT ( 'NONE', #15695 ) ;
#21341=ORIENTED_EDGE ( 'NONE', *, *, #15986, .F. ) ;
#21372=LINE ( 'NONE', #6392, #29920 ) ;
#21408=ORIENTED_EDGE ( 'NONE', *, *, #27494, .F. ) ;
#21463=EDGE_CURVE ( 'NONE', #51023, #44188, #13548, .T. ) ;
#21466=EDGE_CURVE ( 'NONE', #1126, #25732, #22731, .T. ) ;
#21467=ORIENTED_EDGE ( 'NONE', *, *, #39598, .F. ) ;
#21479=ORIENTED_EDGE ( 'NONE', *, *, #44471, .T. ) ;
#21554=EDGE_LOOP ( 'NONE', ( #11748, #21479, #21408, #21467 ) ) ;
#21630=AXIS2_PLACEMENT_3D ( 'NONE', #30228, #2096, #26269 ) ;
#21641=CIRCLE ( 'NONE', #51027, 4.999999999999997335 ) ;
#21849=ORIENTED_EDGE ( 'NONE', *, *, #40946, .F. ) ;
#21894=EDGE_CURVE ( 'NONE', #24400, #51107, #21372, .T. ) ;
#21940=CARTESIAN_POINT ( 'NONE',  ( 3.686287386450715076E-15, 20.00000000000000000, -46.00000000000000711 ) ) ;
#22040=FACE_BOUND ( 'NONE', #44042, .T. ) ;
#22089=CARTESIAN_POINT ( 'NONE',  ( -46.00000000000000711, 20.00000000000000000, -51.00000000000000000 ) ) ;
#22195=CIRCLE ( 'NONE', #18002, 4.999999999999997335 ) ;
#22228=VERTEX_POINT ( 'NONE', #40331 ) ;
#22300=EDGE_LOOP ( 'NONE', ( #33043, #3861 ) ) ;
#22389=AXIS2_PLACEMENT_3D ( 'NONE', #27994, #24069, #31164 ) ;
#22394=DIRECTION ( 'NONE',  ( 0.000000000000000000, 0.000000000000000000, 1.000000000000000000 ) ) ;
#22575=FACE_BOUND ( 'NONE', #5691, .T. ) ;
#22588=CARTESIAN_POINT ( 'NONE',  ( 46.00000000000000000, 20.00000000000000000, 0.000000000000000000 ) ) ;
#22647=ORIENTED_EDGE ( 'NONE', *, *, #25952, .T. ) ;
#22671=AXIS2_PLACEMENT_3D ( 'NONE', #11581, #19220, #27342 ) ;
#22717=DIRECTION ( 'NONE',  ( 0.000000000000000000, 0.000000000000000000, -1.000000000000000000 ) ) ;
#22731=LINE ( 'NONE', #14080, #26661 ) ;
#22734=VERTEX_POINT ( 'NONE', #16653 ) ;
#22745=DIRECTION ( 'NONE',  ( -0.000000000000000000, -1.000000000000000000, -0.000000000000000000 ) ) ;
#22746=DIRECTION ( 'NONE',  ( 0.000000000000000000, 0.000000000000000000, 1.000000000000000000 ) ) ;
#22830=AXIS2_PLACEMENT_3D ( 'NONE', #34500, #14287, #5636 ) ;
#22836=DIRECTION ( 'NONE',  ( 0.000000000000000000, 0.000000000000000000, -1.000000000000000000 ) ) ;
#22841=DIRECTION ( 'NONE',  ( 0.000000000000000000, 1.000000000000000000, 0.000000000000000000 ) ) ;
#22986=LINE ( 'NONE', #6133, #2988 ) ;
#23003=DIRECTION ( 'NONE',  ( 0.000000000000000000, 1.000000000000000000, 0.000000000000000000 ) ) ;
#23006=DIRECTION ( 'NONE',  ( 0.000000000000000000, 0.000000000000000000, 1.000000000000000000 ) ) ;
#23025=EDGE_LOOP ( 'NONE', ( #49902, #643, #23070, #19959 ) ) ;
#23070=ORIENTED_EDGE ( 'NONE', *, *, #29523, .F. ) ;
#23075=VERTEX_POINT ( 'NONE', #32718 ) ;
#23194=EDGE_CURVE ( 'NONE', #28946, #44188, #21641, .T. ) ;
#23384=ORIENTED_EDGE ( 'NONE', *, *, #5789, .T. ) ;
#23406=EDGE_CURVE ( 'NONE', #22228, #18767, #25230, .T. ) ;
#23435=DIRECTION ( 'NONE',  ( 0.000000000000000000, 0.000000000000000000, 1.000000000000000000 ) ) ;
#23514=VERTEX_POINT ( 'NONE', #10748 ) ;
#23534=FACE_BOUND ( 'NONE', #14456, .T. ) ;
#23553=EDGE_CURVE ( 'NONE', #31469, #44223, #31755, .T. ) ;
#23614=EDGE_CURVE ( 'NONE', #44188, #28946, #30896, .T. ) ;
#23641=AXIS2_PLACEMENT_3D ( 'NONE', #5827, #13686, #36827 ) ;
#23787=VERTEX_POINT ( 'NONE', #36988 ) ;
#23862=VECTOR ( 'NONE', #37412, 1000.000000000000000 ) ;
#23896=CARTESIAN_POINT ( 'NONE',  ( -46.00000000000000711, 20.00000000000000000, -41.00000000000000000 ) ) ;
#23957=VECTOR ( 'NONE', #47412, 1000.000000000000000 ) ;
#23996=CIRCLE ( 'NONE', #50877, 4.999999999999997335 ) ;
#24012=ORIENTED_EDGE ( 'NONE', *, *, #37476, .F. ) ;
#24030=COLOUR_RGB ( '', 0.66274510, 0.83137255, 0.94901961) ;
#24049=ADVANCED_FACE ( 'NONE', ( #38545 ), #31170, .F. ) ;
#24069=DIRECTION ( 'NONE',  ( 0.000000000000000000, 1.000000000000000000, -0.000000000000000000 ) ) ;
#24105=CARTESIAN_POINT ( 'NONE',  ( -60.00000000000000000, -43.50000000000000000, -0.000000000000000000 ) ) ;
#24178=VECTOR ( 'NONE', #17766, 1000.000000000000000 ) ;
#24183=ORIENTED_EDGE ( 'NONE', *, *, #32435, .F. ) ;
#24187=AXIS2_PLACEMENT_3D ( 'NONE', #11513, #30452, #22836 ) ;
#24213=ORIENTED_EDGE ( 'NONE', *, *, #4147, .T. ) ;
#24248=ORIENTED_EDGE ( 'NONE', *, *, #17098, .F. ) ;
#24337=ORIENTED_EDGE ( 'NONE', *, *, #6734, .T. ) ;
#24343=ADVANCED_FACE ( 'NONE', ( #7516, #26954, #2781, #39031, #43760, #31157, #39549, #23534, #38776, #3042 ), #7765, .F. ) ;
#24400=VERTEX_POINT ( 'NONE', #30908 ) ;
#24472=EDGE_LOOP ( 'NONE', ( #42095, #27924, #50654, #6502 ) ) ;
#24509=EDGE_CURVE ( 'NONE', #39324, #5146, #42373, .T. ) ;
#24513=ORIENTED_EDGE ( 'NONE', *, *, #4414, .T. ) ;
#24579=LINE ( 'NONE', #40596, #7488 ) ;
#24613=LINE ( 'NONE', #40627, #18588 ) ;
#24662=CYLINDRICAL_SURFACE ( 'NONE', #41758, 4.999999999999997335 ) ;
#24689=DIRECTION ( 'NONE',  ( -0.000000000000000000, -1.000000000000000000, -0.000000000000000000 ) ) ;
#24717=DIRECTION ( 'NONE',  ( 0.000000000000000000, 1.000000000000000000, 0.000000000000000000 ) ) ;
#24879=EDGE_CURVE ( 'NONE', #23075, #7125, #44684, .T. ) ;
#24883=AXIS2_PLACEMENT_3D ( 'NONE', #29587, #25399, #956 ) ;
#24914=DIRECTION ( 'NONE',  ( -0.000000000000000000, -1.000000000000000000, -0.000000000000000000 ) ) ;
#24959=VERTEX_POINT ( 'NONE', #37308 ) ;
#25014=EDGE_LOOP ( 'NONE', ( #37263, #19521, #19966, #3568 ) ) ;
#25027=ADVANCED_FACE ( 'NONE', ( #6561 ), #14440, .F. ) ;
#25029=CARTESIAN_POINT ( 'NONE',  ( 1.734723475976807094E-15, 20.00000000000000000, 46.00000000000000711 ) ) ;
#25035=EDGE_LOOP ( 'NONE', ( #39969, #37523, #21849, #35544 ) ) ;
#25151=ORIENTED_EDGE ( 'NONE', *, *, #38474, .T. ) ;
#25189=DIRECTION ( 'NONE',  ( 0.000000000000000000, 0.000000000000000000, -1.000000000000000000 ) ) ;
#25220=LINE ( 'NONE', #8665, #48607 ) ;
#25230=LINE ( 'NONE', #1580, #4040 ) ;
#25346=DIRECTION ( 'NONE',  ( 0.000000000000000000, 1.000000000000000000, 0.000000000000000000 ) ) ;
#25353=ORIENTED_EDGE ( 'NONE', *, *, #34896, .T. ) ;
#25372=ORIENTED_EDGE ( 'NONE', *, *, #1921, .F. ) ;
#25399=DIRECTION ( 'NONE',  ( -0.000000000000000000, -1.000000000000000000, -0.000000000000000000 ) ) ;
#25438=CIRCLE ( 'NONE', #47281, 4.999999999999997335 ) ;
#25479=ADVANCED_FACE ( 'NONE', ( #4073 ), #7497, .F. ) ;
#25597=EDGE_CURVE ( 'NONE', #5146, #39324, #37424, .T. ) ;
#25730=FACE_BOUND ( 'NONE', #44458, .T. ) ;
#25732=VERTEX_POINT ( 'NONE', #33985 ) ;
#25744=VERTEX_POINT ( 'NONE', #26869 ) ;
#25842=EDGE_CURVE ( 'NONE', #25744, #22228, #47895, .T. ) ;
#25890=PRODUCT_DEFINITION_FORMATION_WITH_SPECIFIED_SOURCE ( 'ANY', '', #5888, .NOT_KNOWN. ) ;
#25895=DIRECTION ( 'NONE',  ( -0.000000000000000000, -1.000000000000000000, -0.000000000000000000 ) ) ;
#25952=EDGE_CURVE ( 'NONE', #24959, #25744, #20281, .T. ) ;
#25956=EDGE_LOOP ( 'NONE', ( #7557, #50882, #41650, #45332 ) ) ;
#26106=AXIS2_PLACEMENT_3D ( 'NONE', #15277, #26833, #46568 ) ;
#26167=ORIENTED_EDGE ( 'NONE', *, *, #46971, .T. ) ;
#26228=DIRECTION ( 'NONE',  ( 0.000000000000000000, -1.000000000000000000, 0.000000000000000000 ) ) ;
#26250=AXIS2_PLACEMENT_3D ( 'NONE', #47326, #11297, #19212 ) ;
#26269=DIRECTION ( 'NONE',  ( 0.000000000000000000, 0.000000000000000000, -1.000000000000000000 ) ) ;
#26284=VERTEX_POINT ( 'NONE', #19204 ) ;
#26307=DIRECTION ( 'NONE',  ( 0.000000000000000000, 0.000000000000000000, 1.000000000000000000 ) ) ;
#26422=CIRCLE ( 'NONE', #2946, 4.999999999999997335 ) ;
#26471=CIRCLE ( 'NONE', #6348, 4.999999999999997335 ) ;
#26477=CARTESIAN_POINT ( 'NONE',  ( 3.686287386450715076E-15, 20.00000000000000000, -46.00000000000000711 ) ) ;
#26494=EDGE_LOOP ( 'NONE', ( #51385, #37640, #2614, #6247 ) ) ;
#26556=ADVANCED_FACE ( 'NONE', ( #49905, #22575, #25730, #37561, #45985, #22040, #38585, #33610, #5784, #30193 ), #49652, .T. ) ;
#26637=CARTESIAN_POINT ( 'NONE',  ( 2.347046875550483230E-15, 20.00000000000000000, 51.00000000000000711 ) ) ;
#26661=VECTOR ( 'NONE', #25895, 1000.000000000000000 ) ;
#26693=ADVANCED_FACE ( 'NONE', ( #27776 ), #3883, .F. ) ;
#26759=ORIENTED_EDGE ( 'NONE', *, *, #36055, .F. ) ;
#26829=ORIENTED_EDGE ( 'NONE', *, *, #14564, .T. ) ;
#26833=DIRECTION ( 'NONE',  ( 0.000000000000000000, 1.000000000000000000, -0.000000000000000000 ) ) ;
#26869=CARTESIAN_POINT ( 'NONE',  ( -60.00000000000000000, 0.000000000000000000, -60.00000000000000711 ) ) ;
#26946=PLANE ( 'NONE',  #21248 ) ;
#26954=FACE_OUTER_BOUND ( 'NONE', #41091, .T. ) ;
#27022=ORIENTED_EDGE ( 'NONE', *, *, #5754, .T. ) ;
#27246=DIRECTION ( 'NONE',  ( 0.000000000000000000, 0.000000000000000000, -1.000000000000000000 ) ) ;
#27287=AXIS2_PLACEMENT_3D ( 'NONE', #19932, #22841, #30712 ) ;
#27310=AXIS2_PLACEMENT_3D ( 'NONE', #1346, #1620, #37344 ) ;
#27342=DIRECTION ( 'NONE',  ( 0.000000000000000000, 0.000000000000000000, -1.000000000000000000 ) ) ;
#27343=ORIENTED_EDGE ( 'NONE', *, *, #40946, .T. ) ;
#27355=DIRECTION ( 'NONE',  ( 0.000000000000000000, 1.000000000000000000, 0.000000000000000000 ) ) ;
#27380=CARTESIAN_POINT ( 'NONE',  ( -46.00000000000000711, 20.00000000000000000, 8.673617379884035472E-15 ) ) ;
#27463=VECTOR ( 'NONE', #29213, 1000.000000000000000 ) ;
#27489=CARTESIAN_POINT ( 'NONE',  ( 3.686287386450715076E-15, 20.00000000000000000, -51.00000000000000711 ) ) ;
#27494=EDGE_CURVE ( 'NONE', #13896, #47167, #21185, .T. ) ;
#27510=ORIENTED_EDGE ( 'NONE', *, *, #17172, .F. ) ;
#27551=EDGE_CURVE ( 'NONE', #41331, #23075, #1030, .T. ) ;
#27560=EDGE_LOOP ( 'NONE', ( #9733, #31265 ) ) ;
#27565=ORIENTED_EDGE ( 'NONE', *, *, #41081, .F. ) ;
#27591=AXIS2_PLACEMENT_3D ( 'NONE', #47466, #7264, #15420 ) ;
#27597=ORIENTED_EDGE ( 'NONE', *, *, #17945, .F. ) ;
#27639=DIRECTION ( 'NONE',  ( -0.000000000000000000, -1.000000000000000000, -0.000000000000000000 ) ) ;
#27689=DIRECTION ( 'NONE',  ( -0.000000000000000000, -0.000000000000000000, 1.000000000000000000 ) ) ;
#27691=EDGE_CURVE ( 'NONE', #40958, #28668, #9407, .T. ) ;
#27776=FACE_OUTER_BOUND ( 'NONE', #28878, .T. ) ;
#27796=AXIS2_PLACEMENT_3D ( 'NONE', #39017, #38520, #23006 ) ;
#27805=EDGE_LOOP ( 'NONE', ( #7149, #31348 ) ) ;
#27814=ORIENTED_EDGE ( 'NONE', *, *, #5754, .F. ) ;
#27838=LINE ( 'NONE', #39658, #38343 ) ;
#27897=DIRECTION ( 'NONE',  ( 0.000000000000000000, 1.000000000000000000, 0.000000000000000000 ) ) ;
#27924=ORIENTED_EDGE ( 'NONE', *, *, #36055, .T. ) ;
#27985=DIRECTION ( 'NONE',  ( 1.000000000000000000, -0.000000000000000000, 0.000000000000000000 ) ) ;
#27994=CARTESIAN_POINT ( 'NONE',  ( -46.00000000000000711, 20.00000000000000000, -46.00000000000000000 ) ) ;
#28030=AXIS2_PLACEMENT_3D ( 'NONE', #11742, #20668, #40120 ) ;
#28137=EDGE_CURVE ( 'NONE', #25732, #26284, #15332, .T. ) ;
#28158=DIRECTION ( 'NONE',  ( 0.000000000000000000, 0.000000000000000000, 1.000000000000000000 ) ) ;
#28200=ORIENTED_EDGE ( 'NONE', *, *, #27691, .F. ) ;
#28226=DIRECTION ( 'NONE',  ( -0.000000000000000000, -1.000000000000000000, -0.000000000000000000 ) ) ;
#28323=AXIS2_PLACEMENT_3D ( 'NONE', #19854, #51938, #36925 ) ;
#28377=ORIENTED_EDGE ( 'NONE', *, *, #25597, .T. ) ;
#28477=ADVANCED_FACE ( 'NONE', ( #49796 ), #13780, .F. ) ;
#28503=VERTEX_POINT ( 'NONE', #38470 ) ;
#28627=VECTOR ( 'NONE', #37624, 1000.000000000000000 ) ;
#28633=AXIS2_PLACEMENT_3D ( 'NONE', #19908, #35939, #14674 ) ;
#28662=VECTOR ( 'NONE', #31397, 1000.000000000000000 ) ;
#28668=VERTEX_POINT ( 'NONE', #44482 ) ;
#28767=DIRECTION ( 'NONE',  ( -5.782411586589357392E-17, 0.000000000000000000, 1.000000000000000000 ) ) ;
#28849=FACE_OUTER_BOUND ( 'NONE', #30787, .T. ) ;
#28878=EDGE_LOOP ( 'NONE', ( #5895, #49556, #41194, #5593 ) ) ;
#28946=VERTEX_POINT ( 'NONE', #38405 ) ;
#28994=VECTOR ( 'NONE', #49968, 1000.000000000000000 ) ;
#29099=CARTESIAN_POINT ( 'NONE',  ( 46.00000000000000000, 20.00000000000000000, -4.999999999999997335 ) ) ;
#29213=DIRECTION ( 'NONE',  ( -0.000000000000000000, -1.000000000000000000, -0.000000000000000000 ) ) ;
#29293=ADVANCED_FACE ( 'NONE', ( #48801 ), #8332, .F. ) ;
#29481=CARTESIAN_POINT ( 'NONE',  ( 0.000000000000000000, -63.50000000000000000, 60.00000000000000711 ) ) ;
#29523=EDGE_CURVE ( 'NONE', #51107, #14767, #45689, .T. ) ;
#29577=ORIENTED_EDGE ( 'NONE', *, *, #1637, .F. ) ;
#29581=ADVANCED_FACE ( 'NONE', ( #42723 ), #34810, .F. ) ;
#29587=CARTESIAN_POINT ( 'NONE',  ( -46.00000000000000711, 20.00000000000000000, -46.00000000000000000 ) ) ;
#29730=EDGE_CURVE ( 'NONE', #51023, #32303, #22195, .T. ) ;
#29774=CARTESIAN_POINT ( 'NONE',  ( 0.000000000000000000, -63.50000000000000000, 20.00000000000000000 ) ) ;
#29775=FACE_OUTER_BOUND ( 'NONE', #26494, .T. ) ;
#29778=PLANE ( 'NONE',  #50751 ) ;
#29797=CARTESIAN_POINT ( 'NONE',  ( 0.000000000000000000, -63.50000000000000000, 0.000000000000000000 ) ) ;
#29817=ADVANCED_FACE ( 'NONE', ( #21124 ), #29778, .T. ) ;
#29822=EDGE_CURVE ( 'NONE', #32303, #28946, #48995, .T. ) ;
#29920=VECTOR ( 'NONE', #14016, 1000.000000000000000 ) ;
#29955=EDGE_LOOP ( 'NONE', ( #43591, #49287, #45468, #21341 ) ) ;
#29978=PRESENTATION_STYLE_ASSIGNMENT (( #13953 ) ) ;
#29982=( LENGTH_UNIT ( ) NAMED_UNIT ( * ) SI_UNIT ( .MILLI., .METRE. ) );
#30010=ORIENTED_EDGE ( 'NONE', *, *, #2477, .F. ) ;
#30078=EDGE_LOOP ( 'NONE', ( #6548, #3641, #4079, #30010 ) ) ;
#30101=ORIENTED_EDGE ( 'NONE', *, *, #23406, .T. ) ;
#30113=DIRECTION ( 'NONE',  ( 0.000000000000000000, 0.000000000000000000, 1.000000000000000000 ) ) ;
#30163=EDGE_CURVE ( 'NONE', #7450, #5492, #44999, .T. ) ;
#30164=CARTESIAN_POINT ( 'NONE',  ( 3.686287386450715076E-15, 20.00000000000000000, -46.00000000000000711 ) ) ;
#30173=ADVANCED_FACE ( 'NONE', ( #8716, #36571 ), #8988, .T. ) ;
#30193=FACE_BOUND ( 'NONE', #8412, .T. ) ;
#30228=CARTESIAN_POINT ( 'NONE',  ( 0.000000000000000000, 20.00000000000000355, 0.000000000000000000 ) ) ;
#30271=VERTEX_POINT ( 'NONE', #38584 ) ;
#30400=ORIENTED_EDGE ( 'NONE', *, *, #37169, .F. ) ;
#30402=CARTESIAN_POINT ( 'NONE',  ( 1.734723475976807094E-15, 0.000000000000000000, 46.00000000000000711 ) ) ;
#30408=DIRECTION ( 'NONE',  ( -0.000000000000000000, -1.000000000000000000, -0.000000000000000000 ) ) ;
#30452=DIRECTION ( 'NONE',  ( 0.000000000000000000, -1.000000000000000000, 0.000000000000000000 ) ) ;
#30462=ORIENTED_EDGE ( 'NONE', *, *, #29523, .T. ) ;
#30507=ORIENTED_EDGE ( 'NONE', *, *, #902, .T. ) ;
#30523=DIRECTION ( 'NONE',  ( 0.000000000000000000, 1.000000000000000000, 0.000000000000000000 ) ) ;
#30584=DIRECTION ( 'NONE',  ( -0.000000000000000000, -1.000000000000000000, -0.000000000000000000 ) ) ;
#30609=CARTESIAN_POINT ( 'NONE',  ( -46.00000000000000711, 0.000000000000000000, 46.00000000000000000 ) ) ;
#30712=DIRECTION ( 'NONE',  ( 0.000000000000000000, 0.000000000000000000, 1.000000000000000000 ) ) ;
#30728=ORIENTED_EDGE ( 'NONE', *, *, #29822, .T. ) ;
#30787=EDGE_LOOP ( 'NONE', ( #49107, #16304, #31575, #1322 ) ) ;
#30896=CIRCLE ( 'NONE', #16655, 4.999999999999997335 ) ;
#30908=CARTESIAN_POINT ( 'NONE',  ( -46.00000000000000711, 20.00000000000000000, 41.00000000000000000 ) ) ;
#30919=VECTOR ( 'NONE', #11924, 1000.000000000000000 ) ;
#31008=ORIENTED_EDGE ( 'NONE', *, *, #39458, .F. ) ;
#31044=ADVANCED_FACE ( 'NONE', ( #1690 ), #5650, .F. ) ;
#31070=FACE_OUTER_BOUND ( 'NONE', #30078, .T. ) ;
#31142=ADVANCED_FACE ( 'NONE', ( #34264 ), #11107, .T. ) ;
#31157=FACE_BOUND ( 'NONE', #46177, .T. ) ;
#31164=DIRECTION ( 'NONE',  ( 0.000000000000000000, 0.000000000000000000, -1.000000000000000000 ) ) ;
#31170=CYLINDRICAL_SURFACE ( 'NONE', #27591, 4.999999999999997335 ) ;
#31172=AXIS2_PLACEMENT_3D ( 'NONE', #29481, #12930, #17155 ) ;
#31192=VERTEX_POINT ( 'NONE', #26637 ) ;
#31265=ORIENTED_EDGE ( 'NONE', *, *, #29730, .F. ) ;
#31276=CYLINDRICAL_SURFACE ( 'NONE', #26250, 4.999999999999997335 ) ;
#31337=CARTESIAN_POINT ( 'NONE',  ( 1.734723475976807094E-15, 0.000000000000000000, 41.00000000000000711 ) ) ;
#31348=ORIENTED_EDGE ( 'NONE', *, *, #39458, .T. ) ;
#31397=DIRECTION ( 'NONE',  ( 1.000000000000000000, -0.000000000000000000, 0.000000000000000000 ) ) ;
#31400=ADVANCED_FACE ( 'NONE', ( #16551 ), #15505, .F. ) ;
#31403=VERTEX_POINT ( 'NONE', #35454 ) ;
#31469=VERTEX_POINT ( 'NONE', #47828 ) ;
#31471=CIRCLE ( 'NONE', #49951, 4.999999999999997335 ) ;
#31482=EDGE_CURVE ( 'NONE', #4347, #39696, #32562, .T. ) ;
#31512=CARTESIAN_POINT ( 'NONE',  ( 60.00000000000001421, 0.000000000000000000, 60.00000000000000711 ) ) ;
#31575=ORIENTED_EDGE ( 'NONE', *, *, #35489, .T. ) ;
#31583=EDGE_LOOP ( 'NONE', ( #17805, #24337, #36945, #11963 ) ) ;
#31631=UNCERTAINTY_MEASURE_WITH_UNIT (LENGTH_MEASURE( 1.000000000000000082E-05 ), #33419, 'distance_accuracy_value', 'NONE');
#31639=CIRCLE ( 'NONE', #35842, 4.999999999999997335 ) ;
#31648=CARTESIAN_POINT ( 'NONE',  ( 30.00000000000000711, -43.50000000000000000, 30.00000000000000355 ) ) ;
#31675=CARTESIAN_POINT ( 'NONE',  ( 0.000000000000000000, -43.50000000000000000, -60.00000000000000711 ) ) ;
#31677=ORIENTED_EDGE ( 'NONE', *, *, #14581, .T. ) ;
#31742=AXIS2_PLACEMENT_3D ( 'NONE', #3714, #31843, #8438 ) ;
#31755=CIRCLE ( 'NONE', #24187, 20.00000000000000000 ) ;
#31809=ORIENTED_EDGE ( 'NONE', *, *, #11718, .T. ) ;
#31843=DIRECTION ( 'NONE',  ( 0.000000000000000000, 0.000000000000000000, 1.000000000000000000 ) ) ;
#31858=CARTESIAN_POINT ( 'NONE',  ( -30.00000000000000000, -43.50000000000000000, -0.000000000000000000 ) ) ;
#31993=EDGE_CURVE ( 'NONE', #36416, #36764, #17718, .T. ) ;
#32009=ORIENTED_EDGE ( 'NONE', *, *, #29730, .T. ) ;
#32022=VERTEX_POINT ( 'NONE', #29774 ) ;
#32097=AXIS2_PLACEMENT_3D ( 'NONE', #38128, #2131, #26307 ) ;
#32156=ORIENTED_EDGE ( 'NONE', *, *, #35489, .F. ) ;
#32226=PLANE ( 'NONE',  #47263 ) ;
#32303=VERTEX_POINT ( 'NONE', #48676 ) ;
#32309=FACE_OUTER_BOUND ( 'NONE', #2982, .T. ) ;
#32349=VECTOR ( 'NONE', #40991, 1000.000000000000000 ) ;
#32399=ORIENTED_EDGE ( 'NONE', *, *, #25597, .F. ) ;
#32421=DIRECTION ( 'NONE',  ( -0.000000000000000000, -1.000000000000000000, -0.000000000000000000 ) ) ;
#32435=EDGE_CURVE ( 'NONE', #31403, #36384, #38117, .T. ) ;
#32461=PLANE ( 'NONE',  #28323 ) ;
#32562=LINE ( 'NONE', #48612, #7111 ) ;
#32718=CARTESIAN_POINT ( 'NONE',  ( -46.00000000000000711, 20.00000000000000000, -4.999999999999988454 ) ) ;
#32735=EDGE_CURVE ( 'NONE', #21250, #26284, #39655, .T. ) ;
#32881=CARTESIAN_POINT ( 'NONE',  ( 0.000000000000000000, -63.50000000000000000, 0.000000000000000000 ) ) ;
#32884=VECTOR ( 'NONE', #47655, 1000.000000000000000 ) ;
#32902=CARTESIAN_POINT ( 'NONE',  ( 46.00000000000000711, 20.00000000000000000, 41.00000000000000000 ) ) ;
#32978=CARTESIAN_POINT ( 'NONE',  ( -46.00000000000000711, 20.00000000000000000, 5.000000000000006217 ) ) ;
#33031=CARTESIAN_POINT ( 'NONE',  ( -46.00000000000000711, 20.00000000000000000, 8.673617379884035472E-15 ) ) ;
#33043=ORIENTED_EDGE ( 'NONE', *, *, #37236, .F. ) ;
#33075=ORIENTED_EDGE ( 'NONE', *, *, #4414, .F. ) ;
#33121=ORIENTED_EDGE ( 'NONE', *, *, #9124, .F. ) ;
#33132=EDGE_LOOP ( 'NONE', ( #51816, #24183, #13246, #46991 ) ) ;
#33134=( NAMED_UNIT ( * ) PLANE_ANGLE_UNIT ( ) SI_UNIT ( $, .RADIAN. ) );
#33263=VECTOR ( 'NONE', #46232, 1000.000000000000000 ) ;
#33270=AXIS2_PLACEMENT_3D ( 'NONE', #7093, #3397, #39639 ) ;
#33419=( LENGTH_UNIT ( ) NAMED_UNIT ( * ) SI_UNIT ( .MILLI., .METRE. ) );
#33454=FACE_OUTER_BOUND ( 'NONE', #469, .T. ) ;
#33541=ORIENTED_EDGE ( 'NONE', *, *, #37476, .T. ) ;
#33548=FACE_OUTER_BOUND ( 'NONE', #12645, .T. ) ;
#33587=DIRECTION ( 'NONE',  ( 1.000000000000000000, 0.000000000000000000, 0.000000000000000000 ) ) ;
#33610=FACE_BOUND ( 'NONE', #27805, .T. ) ;
#33694=CARTESIAN_POINT ( 'NONE',  ( 0.000000000000000000, -63.50000000000000000, 20.00000000000000000 ) ) ;
#33728=EDGE_LOOP ( 'NONE', ( #35419, #40870, #7547, #24513 ) ) ;
#33743=LINE ( 'NONE', #45840, #11051 ) ;
#33765=VECTOR ( 'NONE', #1796, 1000.000000000000000 ) ;
#33812=EDGE_CURVE ( 'NONE', #2088, #33816, #20042, .T. ) ;
#33816=VERTEX_POINT ( 'NONE', #35809 ) ;
#33985=CARTESIAN_POINT ( 'NONE',  ( -46.00000000000000711, 0.000000000000000000, -51.00000000000000000 ) ) ;
#33995=DIRECTION ( 'NONE',  ( -0.000000000000000000, -1.000000000000000000, -0.000000000000000000 ) ) ;
#34023=FACE_OUTER_BOUND ( 'NONE', #25014, .T. ) ;
#34153=CARTESIAN_POINT ( 'NONE',  ( 46.00000000000000000, 0.000000000000000000, -4.999999999999997335 ) ) ;
#34168=LINE ( 'NONE', #6058, #45185 ) ;
#34214=EDGE_LOOP ( 'NONE', ( #4770, #26167, #28200, #20958 ) ) ;
#34227=EDGE_CURVE ( 'NONE', #26284, #25732, #40066, .T. ) ;
#34249=CARTESIAN_POINT ( 'NONE',  ( -60.00000000000000000, -63.50000000000000000, -60.00000000000000711 ) ) ;
#34253=ADVANCED_FACE ( 'NONE', ( #40853 ), #32461, .F. ) ;
#34264=FACE_OUTER_BOUND ( 'NONE', #14554, .T. ) ;
#34356=ORIENTED_EDGE ( 'NONE', *, *, #43874, .T. ) ;
#34364=CARTESIAN_POINT ( 'NONE',  ( -46.00000000000000711, 20.00000000000000000, 5.000000000000006217 ) ) ;
#34411=LINE ( 'NONE', #50707, #5781 ) ;
#34446=CARTESIAN_POINT ( 'NONE',  ( 30.00000000000000711, -43.50000000000000000, -30.00000000000000355 ) ) ;
#34478=ORIENTED_EDGE ( 'NONE', *, *, #29822, .F. ) ;
#34500=CARTESIAN_POINT ( 'NONE',  ( 30.00000000000000711, -43.50000000000000000, 0.000000000000000000 ) ) ;
#34516=ORIENTED_EDGE ( 'NONE', *, *, #45270, .T. ) ;
#34525=EDGE_LOOP ( 'NONE', ( #47242, #19309, #42714, #49154 ) ) ;
#34531=FACE_OUTER_BOUND ( 'NONE', #48201, .T. ) ;
#34560=VECTOR ( 'NONE', #38950, 1000.000000000000000 ) ;
#34564=ORIENTED_EDGE ( 'NONE', *, *, #36192, .F. ) ;
#34644=DIRECTION ( 'NONE',  ( 0.000000000000000000, 1.000000000000000000, -0.000000000000000000 ) ) ;
#34728=ORIENTED_EDGE ( 'NONE', *, *, #14442, .F. ) ;
#34744=EDGE_LOOP ( 'NONE', ( #22647, #27510, #15657, #23384 ) ) ;
#34787=ORIENTED_EDGE ( 'NONE', *, *, #47620, .T. ) ;
#34789=CARTESIAN_POINT ( 'NONE',  ( 1.734723475976807094E-15, 20.00000000000000000, 46.00000000000000711 ) ) ;
#34810=CYLINDRICAL_SURFACE ( 'NONE', #13795, 4.999999999999997335 ) ;
#34849=ORIENTED_EDGE ( 'NONE', *, *, #4819, .F. ) ;
#34868=ORIENTED_EDGE ( 'NONE', *, *, #32735, .F. ) ;
#34896=EDGE_CURVE ( 'NONE', #32022, #44223, #40784, .T. ) ;
#35034=LINE ( 'NONE', #39985, #14531 ) ;
#35066=CARTESIAN_POINT ( 'NONE',  ( 46.00000000000000000, 0.000000000000000000, 0.000000000000000000 ) ) ;
#35271=LINE ( 'NONE', #47891, #14866 ) ;
#35339=DIRECTION ( 'NONE',  ( 0.000000000000000000, 1.000000000000000000, 0.000000000000000000 ) ) ;
#35381=CIRCLE ( 'NONE', #27796, 4.999999999999997335 ) ;
#35390=DIRECTION ( 'NONE',  ( 0.000000000000000000, 0.000000000000000000, 1.000000000000000000 ) ) ;
#35419=ORIENTED_EDGE ( 'NONE', *, *, #49043, .T. ) ;
#35454=CARTESIAN_POINT ( 'NONE',  ( 60.00000000000001421, -63.50000000000000000, -60.00000000000000711 ) ) ;
#35474=DIRECTION ( 'NONE',  ( 0.000000000000000000, 1.000000000000000000, -0.000000000000000000 ) ) ;
#35487=CARTESIAN_POINT ( 'NONE',  ( 30.00000000000000711, 0.000000000000000000, 30.00000000000000355 ) ) ;
#35489=EDGE_CURVE ( 'NONE', #30271, #36384, #3904, .T. ) ;
#35544=ORIENTED_EDGE ( 'NONE', *, *, #6854, .T. ) ;
#35572=VERTEX_POINT ( 'NONE', #984 ) ;
#35652=CARTESIAN_POINT ( 'NONE',  ( -60.00000000000000000, 20.00000000000000000, -60.00000000000000711 ) ) ;
#35759=AXIS2_PLACEMENT_3D ( 'NONE', #20091, #28226, #48217 ) ;
#35809=CARTESIAN_POINT ( 'NONE',  ( -60.00000000000000000, -43.50000000000000000, 60.00000000000000711 ) ) ;
#35833=VECTOR ( 'NONE', #15330, 1000.000000000000000 ) ;
#35842=AXIS2_PLACEMENT_3D ( 'NONE', #18711, #27355, #23435 ) ;
#35866=CARTESIAN_POINT ( 'NONE',  ( 0.000000000000000000, 20.00000000000000355, 20.00000000000000000 ) ) ;
#35939=DIRECTION ( 'NONE',  ( -0.000000000000000000, -1.000000000000000000, -0.000000000000000000 ) ) ;
#35946=( GEOMETRIC_REPRESENTATION_CONTEXT ( 3 ) GLOBAL_UNCERTAINTY_ASSIGNED_CONTEXT ( ( #2740 ) ) GLOBAL_UNIT_ASSIGNED_CONTEXT ( ( #29982, #42313, #46037 ) ) REPRESENTATION_CONTEXT ( 'NONE', 'WORKASPACE' ) );
#35954=ADVANCED_FACE ( 'NONE', ( #44820 ), #49999, .F. ) ;
#36007=ORIENTED_EDGE ( 'NONE', *, *, #10832, .T. ) ;
#36055=EDGE_CURVE ( 'NONE', #7418, #31469, #24579, .T. ) ;
#36142=EDGE_LOOP ( 'NONE', ( #25372, #33121 ) ) ;
#36162=CYLINDRICAL_SURFACE ( 'NONE', #50968, 4.999999999999997335 ) ;
#36192=EDGE_CURVE ( 'NONE', #755, #40102, #2494, .T. ) ;
#36251=AXIS2_PLACEMENT_3D ( 'NONE', #17854, #9982, #5792 ) ;
#36261=CIRCLE ( 'NONE', #32097, 4.999999999999997335 ) ;
#36340=CARTESIAN_POINT ( 'NONE',  ( 30.00000000000000711, -43.50000000000000000, 0.000000000000000000 ) ) ;
#36384=VERTEX_POINT ( 'NONE', #16846 ) ;
#36416=VERTEX_POINT ( 'NONE', #48902 ) ;
#36483=CARTESIAN_POINT ( 'NONE',  ( 30.00000000000000711, 0.000000000000000000, 30.00000000000000355 ) ) ;
#36530=CARTESIAN_POINT ( 'NONE',  ( -60.00000000000000000, -63.50000000000000000, 60.00000000000000711 ) ) ;
#36563=EDGE_CURVE ( 'NONE', #28503, #7450, #34411, .T. ) ;
#36571=FACE_OUTER_BOUND ( 'NONE', #39513, .T. ) ;
#36662=DIRECTION ( 'NONE',  ( 0.000000000000000000, 0.000000000000000000, -1.000000000000000000 ) ) ;
#36764=VERTEX_POINT ( 'NONE', #49363 ) ;
#36773=DIRECTION ( 'NONE',  ( 1.000000000000000000, 0.000000000000000000, 0.000000000000000000 ) ) ;
#36827=DIRECTION ( 'NONE',  ( -1.000000000000000000, 0.000000000000000000, -0.000000000000000000 ) ) ;
#36889=EDGE_LOOP ( 'NONE', ( #40010, #32009, #30728, #49942 ) ) ;
#36892=EDGE_CURVE ( 'NONE', #41489, #40958, #25220, .T. ) ;
#36925=DIRECTION ( 'NONE',  ( 1.000000000000000000, 0.000000000000000000, 0.000000000000000000 ) ) ;
#36945=ORIENTED_EDGE ( 'NONE', *, *, #48869, .F. ) ;
#36959=VECTOR ( 'NONE', #4405, 1000.000000000000000 ) ;
#36966=CYLINDRICAL_SURFACE ( 'NONE', #24883, 4.999999999999997335 ) ;
#36988=CARTESIAN_POINT ( 'NONE',  ( -30.00000000000000000, 0.000000000000000000, 30.00000000000000355 ) ) ;
#37037=CARTESIAN_POINT ( 'NONE',  ( 2.449293598294706119E-15, -63.50000000000000000, -20.00000000000000000 ) ) ;
#37165=CARTESIAN_POINT ( 'NONE',  ( 0.000000000000000000, -63.50000000000000000, 0.000000000000000000 ) ) ;
#37169=EDGE_CURVE ( 'NONE', #14767, #51107, #11671, .T. ) ;
#37173=AXIS2_PLACEMENT_3D ( 'NONE', #44902, #1532, #9166 ) ;
#37236=EDGE_CURVE ( 'NONE', #23075, #41331, #10852, .T. ) ;
#37263=ORIENTED_EDGE ( 'NONE', *, *, #17605, .T. ) ;
#37274=ORIENTED_EDGE ( 'NONE', *, *, #23194, .T. ) ;
#37308=CARTESIAN_POINT ( 'NONE',  ( 60.00000000000001421, 0.000000000000000000, -60.00000000000000711 ) ) ;
#37344=DIRECTION ( 'NONE',  ( 0.000000000000000000, 0.000000000000000000, -1.000000000000000000 ) ) ;
#37412=DIRECTION ( 'NONE',  ( -0.000000000000000000, -1.000000000000000000, -0.000000000000000000 ) ) ;
#37424=CIRCLE ( 'NONE', #500, 4.999999999999997335 ) ;
#37476=EDGE_CURVE ( 'NONE', #5492, #23514, #18045, .T. ) ;
#37523=ORIENTED_EDGE ( 'NONE', *, *, #43648, .F. ) ;
#37548=DIRECTION ( 'NONE',  ( 0.000000000000000000, 1.000000000000000000, 0.000000000000000000 ) ) ;
#37552=LINE ( 'NONE', #18094, #33765 ) ;
#37561=FACE_BOUND ( 'NONE', #9268, .T. ) ;
#37600=DIRECTION ( 'NONE',  ( 1.000000000000000000, -0.000000000000000000, 0.000000000000000000 ) ) ;
#37609=EDGE_CURVE ( 'NONE', #36764, #36384, #16439, .T. ) ;
#37623=CARTESIAN_POINT ( 'NONE',  ( 60.00000000000001421, -63.50000000000000000, -60.00000000000000711 ) ) ;
#37624=DIRECTION ( 'NONE',  ( 0.000000000000000000, 1.000000000000000000, 0.000000000000000000 ) ) ;
#37640=ORIENTED_EDGE ( 'NONE', *, *, #18949, .F. ) ;
#37672=EDGE_LOOP ( 'NONE', ( #43996, #38841, #15068, #19710 ) ) ;
#37682=DIRECTION ( 'NONE',  ( 0.000000000000000000, 0.000000000000000000, -1.000000000000000000 ) ) ;
#37895=ADVANCED_FACE ( 'NONE', ( #3185 ), #15530, .F. ) ;
#37993=DIRECTION ( 'NONE',  ( 0.000000000000000000, 0.000000000000000000, -1.000000000000000000 ) ) ;
#38011=VERTEX_POINT ( 'NONE', #5265 ) ;
#38082=DIRECTION ( 'NONE',  ( 0.000000000000000000, 0.000000000000000000, -1.000000000000000000 ) ) ;
#38117=LINE ( 'NONE', #37623, #28994 ) ;
#38128=CARTESIAN_POINT ( 'NONE',  ( 46.00000000000000711, 20.00000000000000000, -46.00000000000000000 ) ) ;
#38142=DIRECTION ( 'NONE',  ( -0.000000000000000000, 1.000000000000000000, -0.000000000000000000 ) ) ;
#38161=ORIENTED_EDGE ( 'NONE', *, *, #23614, .T. ) ;
#38191=DIRECTION ( 'NONE',  ( 1.000000000000000000, 0.000000000000000000, 0.000000000000000000 ) ) ;
#38193=ORIENTED_EDGE ( 'NONE', *, *, #43336, .T. ) ;
#38205=CARTESIAN_POINT ( 'NONE',  ( 46.00000000000000711, 0.000000000000000000, -46.00000000000000000 ) ) ;
#38218=DIRECTION ( 'NONE',  ( 0.000000000000000000, 1.000000000000000000, 0.000000000000000000 ) ) ;
#38257=DIRECTION ( 'NONE',  ( -1.000000000000000000, 0.000000000000000000, 0.000000000000000000 ) ) ;
#38319=ORIENTED_EDGE ( 'NONE', *, *, #902, .F. ) ;
#38325=DIRECTION ( 'NONE',  ( 0.000000000000000000, -0.000000000000000000, -1.000000000000000000 ) ) ;
#38343=VECTOR ( 'NONE', #19698, 1000.000000000000000 ) ;
#38405=CARTESIAN_POINT ( 'NONE',  ( 46.00000000000000711, 0.000000000000000000, -51.00000000000000000 ) ) ;
#38470=CARTESIAN_POINT ( 'NONE',  ( 60.00000000000001421, 20.00000000000000000, 60.00000000000000711 ) ) ;
#38474=EDGE_CURVE ( 'NONE', #23514, #22228, #16776, .T. ) ;
#38483=ORIENTED_EDGE ( 'NONE', *, *, #51228, .T. ) ;
#38491=DIRECTION ( 'NONE',  ( 0.000000000000000000, 0.000000000000000000, 1.000000000000000000 ) ) ;
#38504=VECTOR ( 'NONE', #16248, 1000.000000000000000 ) ;
#38520=DIRECTION ( 'NONE',  ( 0.000000000000000000, 1.000000000000000000, 0.000000000000000000 ) ) ;
#38545=FACE_OUTER_BOUND ( 'NONE', #25956, .T. ) ;
#38584=CARTESIAN_POINT ( 'NONE',  ( 60.00000000000001421, -43.50000000000000000, 60.00000000000000711 ) ) ;
#38585=FACE_BOUND ( 'NONE', #43516, .T. ) ;
#38599=ORIENTED_EDGE ( 'NONE', *, *, #11223, .F. ) ;
#38753=VECTOR ( 'NONE', #46276, 1000.000000000000000 ) ;
#38776=FACE_BOUND ( 'NONE', #45232, .T. ) ;
#38841=ORIENTED_EDGE ( 'NONE', *, *, #14442, .T. ) ;
#38950=DIRECTION ( 'NONE',  ( 0.000000000000000000, 0.000000000000000000, -1.000000000000000000 ) ) ;
#38955=CARTESIAN_POINT ( 'NONE',  ( -60.00000000000000000, 20.00000000000000000, -60.00000000000000711 ) ) ;
#38964=ORIENTED_EDGE ( 'NONE', *, *, #44128, .T. ) ;
#39017=CARTESIAN_POINT ( 'NONE',  ( 3.686287386450715076E-15, 0.000000000000000000, -46.00000000000000711 ) ) ;
#39031=FACE_BOUND ( 'NONE', #27560, .T. ) ;
#39033=ORIENTED_EDGE ( 'NONE', *, *, #33812, .T. ) ;
#39289=DIRECTION ( 'NONE',  ( 0.000000000000000000, 0.000000000000000000, -1.000000000000000000 ) ) ;
#39324=VERTEX_POINT ( 'NONE', #32902 ) ;
#39417=ADVANCED_FACE ( 'NONE', ( #33454 ), #48953, .T. ) ;
#39421=DIRECTION ( 'NONE',  ( 0.000000000000000000, 1.000000000000000000, 0.000000000000000000 ) ) ;
#39458=EDGE_CURVE ( 'NONE', #10970, #2101, #15239, .T. ) ;
#39483=CARTESIAN_POINT ( 'NONE',  ( -30.00000000000000000, -43.50000000000000000, -30.00000000000000711 ) ) ;
#39513=EDGE_LOOP ( 'NONE', ( #1686, #26829, #19349, #24248 ) ) ;
#39549=FACE_BOUND ( 'NONE', #36142, .T. ) ;
#39598=EDGE_CURVE ( 'NONE', #40102, #13896, #16515, .T. ) ;
#39604=DIRECTION ( 'NONE',  ( 0.000000000000000000, 0.000000000000000000, 1.000000000000000000 ) ) ;
#39639=DIRECTION ( 'NONE',  ( 0.000000000000000000, 0.000000000000000000, 1.000000000000000000 ) ) ;
#39655=LINE ( 'NONE', #23896, #3882 ) ;
#39658=CARTESIAN_POINT ( 'NONE',  ( 46.00000000000000711, 20.00000000000000000, 41.00000000000000000 ) ) ;
#39696=VERTEX_POINT ( 'NONE', #35487 ) ;
#39756=CARTESIAN_POINT ( 'NONE',  ( -30.00000000000000000, 0.000000000000000000, 30.00000000000000355 ) ) ;
#39918=CARTESIAN_POINT ( 'NONE',  ( -30.00000000000000000, -43.50000000000000000, 30.00000000000000355 ) ) ;
#39925=FACE_OUTER_BOUND ( 'NONE', #31583, .T. ) ;
#39928=CARTESIAN_POINT ( 'NONE',  ( -60.00000000000000000, -63.50000000000000000, 0.000000000000000000 ) ) ;
#39969=ORIENTED_EDGE ( 'NONE', *, *, #4147, .F. ) ;
#39985=CARTESIAN_POINT ( 'NONE',  ( 1.734723475976807489E-15, -43.50000000000000000, -30.00000000000000711 ) ) ;
#40003=EDGE_CURVE ( 'NONE', #41331, #17289, #20918, .T. ) ;
#40010=ORIENTED_EDGE ( 'NONE', *, *, #21463, .F. ) ;
#40066=CIRCLE ( 'NONE', #2313, 4.999999999999997335 ) ;
#40075=CARTESIAN_POINT ( 'NONE',  ( 46.00000000000000711, 20.00000000000000000, 46.00000000000000000 ) ) ;
#40102=VERTEX_POINT ( 'NONE', #1968 ) ;
#40120=DIRECTION ( 'NONE',  ( 0.000000000000000000, 0.000000000000000000, -1.000000000000000000 ) ) ;
#40186=ADVANCED_FACE ( 'NONE', ( #34531 ), #51608, .F. ) ;
#40203=PLANE ( 'NONE',  #51405 ) ;
#40269=DIRECTION ( 'NONE',  ( 0.000000000000000000, 0.000000000000000000, -1.000000000000000000 ) ) ;
#40314=ORIENTED_EDGE ( 'NONE', *, *, #44163, .T. ) ;
#40331=CARTESIAN_POINT ( 'NONE',  ( -60.00000000000000000, 0.000000000000000000, 60.00000000000000711 ) ) ;
#40352=ORIENTED_EDGE ( 'NONE', *, *, #31993, .F. ) ;
#40378=DIRECTION ( 'NONE',  ( 0.000000000000000000, 0.000000000000000000, 1.000000000000000000 ) ) ;
#40398=ADVANCED_FACE ( 'NONE', ( #39925 ), #31276, .F. ) ;
#40428=CARTESIAN_POINT ( 'NONE',  ( 4.298610786024391605E-15, 20.00000000000000000, -41.00000000000000711 ) ) ;
#40450=DIRECTION ( 'NONE',  ( 0.000000000000000000, 0.000000000000000000, 1.000000000000000000 ) ) ;
#40596=CARTESIAN_POINT ( 'NONE',  ( 2.449293598294706119E-15, -63.50000000000000000, -20.00000000000000000 ) ) ;
#40627=CARTESIAN_POINT ( 'NONE',  ( 60.00000000000001421, -63.50000000000000000, 0.000000000000000000 ) ) ;
#40673=CARTESIAN_POINT ( 'NONE',  ( 46.00000000000000711, 20.00000000000000000, -46.00000000000000000 ) ) ;
#40784=LINE ( 'NONE', #33694, #42668 ) ;
#40853=FACE_OUTER_BOUND ( 'NONE', #33132, .T. ) ;
#40870=ORIENTED_EDGE ( 'NONE', *, *, #5789, .F. ) ;
#40946=EDGE_CURVE ( 'NONE', #51787, #48702, #35034, .T. ) ;
#40958=VERTEX_POINT ( 'NONE', #31337 ) ;
#40991=DIRECTION ( 'NONE',  ( -0.000000000000000000, -1.000000000000000000, -0.000000000000000000 ) ) ;
#41010=EDGE_CURVE ( 'NONE', #41489, #31192, #43884, .T. ) ;
#41027=FACE_OUTER_BOUND ( 'NONE', #18244, .T. ) ;
#41081=EDGE_CURVE ( 'NONE', #40102, #755, #25438, .T. ) ;
#41091=EDGE_LOOP ( 'NONE', ( #18409, #48599, #33541, #47442 ) ) ;
#41099=DIRECTION ( 'NONE',  ( 0.000000000000000000, 1.000000000000000000, -0.000000000000000000 ) ) ;
#41108=APPLICATION_CONTEXT ( 'automotive_design' ) ;
#41188=ADVANCED_FACE ( 'NONE', ( #4693, #28849 ), #20453, .F. ) ;
#41194=ORIENTED_EDGE ( 'NONE', *, *, #28137, .F. ) ;
#41244=DIRECTION ( 'NONE',  ( 1.000000000000000000, 0.000000000000000000, 0.000000000000000000 ) ) ;
#41255=ORIENTED_EDGE ( 'NONE', *, *, #32435, .T. ) ;
#41274=FILL_AREA_STYLE_COLOUR ( '', #24030 ) ;
#41331=VERTEX_POINT ( 'NONE', #34364 ) ;
#41370=AXIS2_PLACEMENT_3D ( 'NONE', #25029, #44473, #1090 ) ;
#41422=ORIENTED_EDGE ( 'NONE', *, *, #34227, .T. ) ;
#41489=VERTEX_POINT ( 'NONE', #47487 ) ;
#41526=FACE_OUTER_BOUND ( 'NONE', #7126, .T. ) ;
#41550=DIRECTION ( 'NONE',  ( 0.000000000000000000, 1.000000000000000000, 0.000000000000000000 ) ) ;
#41650=ORIENTED_EDGE ( 'NONE', *, *, #14164, .F. ) ;
#41718=DIRECTION ( 'NONE',  ( 0.000000000000000000, 0.000000000000000000, 1.000000000000000000 ) ) ;
#41758=AXIS2_PLACEMENT_3D ( 'NONE', #40673, #16802, #48856 ) ;
#41779=DIRECTION ( 'NONE',  ( -0.000000000000000000, -1.000000000000000000, -0.000000000000000000 ) ) ;
#41893=ORIENTED_EDGE ( 'NONE', *, *, #14164, .T. ) ;
#41895=DIRECTION ( 'NONE',  ( 0.000000000000000000, 0.000000000000000000, 1.000000000000000000 ) ) ;
#41923=DIRECTION ( 'NONE',  ( -0.000000000000000000, -1.000000000000000000, -0.000000000000000000 ) ) ;
#41927=CARTESIAN_POINT ( 'NONE',  ( -30.00000000000000000, 0.000000000000000000, -30.00000000000000711 ) ) ;
#41940=CARTESIAN_POINT ( 'NONE',  ( -46.00000000000000711, 20.00000000000000000, 46.00000000000000000 ) ) ;
#42095=ORIENTED_EDGE ( 'NONE', *, *, #7025, .F. ) ;
#42201=CARTESIAN_POINT ( 'NONE',  ( -60.00000000000000000, 20.00000000000000000, 60.00000000000000711 ) ) ;
#42299=ORIENTED_EDGE ( 'NONE', *, *, #17605, .F. ) ;
#42313=( NAMED_UNIT ( * ) PLANE_ANGLE_UNIT ( ) SI_UNIT ( $, .RADIAN. ) );
#42338=AXIS2_PLACEMENT_3D ( 'NONE', #35066, #38218, #38491 ) ;
#42359=LINE ( 'NONE', #11070, #46542 ) ;
#42373=CIRCLE ( 'NONE', #9671, 4.999999999999997335 ) ;
#42400=ORIENTED_EDGE ( 'NONE', *, *, #6734, .F. ) ;
#42666=LINE ( 'NONE', #39483, #32884 ) ;
#42668=VECTOR ( 'NONE', #49732, 1000.000000000000000 ) ;
#42714=ORIENTED_EDGE ( 'NONE', *, *, #25842, .F. ) ;
#42723=FACE_OUTER_BOUND ( 'NONE', #34214, .T. ) ;
#43222=VECTOR ( 'NONE', #50294, 1000.000000000000000 ) ;
#43285=DIRECTION ( 'NONE',  ( 1.000000000000000000, 0.000000000000000000, -0.000000000000000000 ) ) ;
#43308=DIRECTION ( 'NONE',  ( 0.000000000000000000, 1.000000000000000000, 0.000000000000000000 ) ) ;
#43320=DIRECTION ( 'NONE',  ( 0.000000000000000000, 1.000000000000000000, 0.000000000000000000 ) ) ;
#43324=ADVANCED_FACE ( 'NONE', ( #29775 ), #49524, .T. ) ;
#43336=EDGE_CURVE ( 'NONE', #6145, #51787, #19504, .T. ) ;
#43432=DIRECTION ( 'NONE',  ( -0.000000000000000000, -1.000000000000000000, -0.000000000000000000 ) ) ;
#43516=EDGE_LOOP ( 'NONE', ( #37274, #38161 ) ) ;
#43527=VECTOR ( 'NONE', #32421, 1000.000000000000000 ) ;
#43540=DIRECTION ( 'NONE',  ( 0.000000000000000000, 1.000000000000000000, 0.000000000000000000 ) ) ;
#43591=ORIENTED_EDGE ( 'NONE', *, *, #44471, .F. ) ;
#43603=ORIENTED_EDGE ( 'NONE', *, *, #8551, .F. ) ;
#43640=EDGE_LOOP ( 'NONE', ( #6707, #13636, #12271, #34478 ) ) ;
#43648=EDGE_CURVE ( 'NONE', #48702, #15921, #10276, .T. ) ;
#43677=LINE ( 'NONE', #8393, #46348 ) ;
#43760=FACE_BOUND ( 'NONE', #11638, .T. ) ;
#43874=EDGE_CURVE ( 'NONE', #14462, #31403, #24613, .T. ) ;
#43884=CIRCLE ( 'NONE', #41370, 4.999999999999997335 ) ;
#43996=ORIENTED_EDGE ( 'NONE', *, *, #46971, .F. ) ;
#44042=EDGE_LOOP ( 'NONE', ( #31809, #3127, #24213, #31677 ) ) ;
#44128=EDGE_CURVE ( 'NONE', #38011, #12927, #35381, .T. ) ;
#44163=EDGE_CURVE ( 'NONE', #6145, #4347, #7503, .T. ) ;
#44172=AXIS2_PLACEMENT_3D ( 'NONE', #37165, #25346, #905 ) ;
#44180=CIRCLE ( 'NONE', #33270, 4.999999999999997335 ) ;
#44188=VERTEX_POINT ( 'NONE', #4080 ) ;
#44223=VERTEX_POINT ( 'NONE', #35866 ) ;
#44338=ORIENTED_EDGE ( 'NONE', *, *, #15986, .T. ) ;
#44398=CARTESIAN_POINT ( 'NONE',  ( 30.00000000000000711, -43.50000000000000000, -30.00000000000000355 ) ) ;
#44458=EDGE_LOOP ( 'NONE', ( #17567, #41422 ) ) ;
#44471=EDGE_CURVE ( 'NONE', #755, #47167, #4244, .T. ) ;
#44473=DIRECTION ( 'NONE',  ( 0.000000000000000000, 1.000000000000000000, 0.000000000000000000 ) ) ;
#44476=CARTESIAN_POINT ( 'NONE',  ( 0.000000000000000000, -63.50000000000000000, 0.000000000000000000 ) ) ;
#44482=CARTESIAN_POINT ( 'NONE',  ( 2.347046875550483230E-15, 0.000000000000000000, 51.00000000000000711 ) ) ;
#44495=LINE ( 'NONE', #36340, #45964 ) ;
#44515=LINE ( 'NONE', #3531, #43527 ) ;
#44518=VECTOR ( 'NONE', #48934, 1000.000000000000000 ) ;
#44563=ORIENTED_EDGE ( 'NONE', *, *, #14581, .F. ) ;
#44587=ADVANCED_FACE ( 'NONE', ( #41526 ), #16862, .F. ) ;
#44597=AXIS2_PLACEMENT_3D ( 'NONE', #17984, #45839, #21132 ) ;
#44633=DIRECTION ( 'NONE',  ( 0.000000000000000000, 1.000000000000000000, -0.000000000000000000 ) ) ;
#44634=EDGE_LOOP ( 'NONE', ( #42400, #28377, #14799, #31008 ) ) ;
#44684=LINE ( 'NONE', #49666, #32349 ) ;
#44701=EDGE_CURVE ( 'NONE', #35572, #14767, #50996, .T. ) ;
#44728=DIRECTION ( 'NONE',  ( -1.000000000000000000, -0.000000000000000000, -0.000000000000000000 ) ) ;
#44782=EDGE_LOOP ( 'NONE', ( #42299, #34849 ) ) ;
#44820=FACE_OUTER_BOUND ( 'NONE', #25035, .T. ) ;
#44902=CARTESIAN_POINT ( 'NONE',  ( 0.000000000000000000, -43.50000000000000000, 0.000000000000000000 ) ) ;
#44999=LINE ( 'NONE', #16878, #12149 ) ;
#45065=CARTESIAN_POINT ( 'NONE',  ( 46.00000000000000711, 20.00000000000000000, -51.00000000000000000 ) ) ;
#45073=ORIENTED_EDGE ( 'NONE', *, *, #21466, .T. ) ;
#45083=AXIS2_PLACEMENT_3D ( 'NONE', #48681, #835, #28158 ) ;
#45185=VECTOR ( 'NONE', #37600, 1000.000000000000000 ) ;
#45232=EDGE_LOOP ( 'NONE', ( #45797, #34728 ) ) ;
#45270=EDGE_CURVE ( 'NONE', #33816, #36764, #20400, .T. ) ;
#45273=ADVANCED_FACE ( 'NONE', ( #16211 ), #32226, .F. ) ;
#45332=ORIENTED_EDGE ( 'NONE', *, *, #24879, .F. ) ;
#45468=ORIENTED_EDGE ( 'NONE', *, *, #39598, .T. ) ;
#45500=( NAMED_UNIT ( * ) SI_UNIT ( $, .STERADIAN. ) SOLID_ANGLE_UNIT ( ) );
#45685=CARTESIAN_POINT ( 'NONE',  ( -30.00000000000000000, 0.000000000000000000, 30.00000000000000355 ) ) ;
#45689=CIRCLE ( 'NONE', #49851, 4.999999999999997335 ) ;
#45759=SHAPE_REPRESENTATION_RELATIONSHIP ( 'NONE' , 'NONE' ,  #15639, #15504 ) ;
#45797=ORIENTED_EDGE ( 'NONE', *, *, #41010, .F. ) ;
#45839=DIRECTION ( 'NONE',  ( -0.000000000000000000, -1.000000000000000000, -0.000000000000000000 ) ) ;
#45840=CARTESIAN_POINT ( 'NONE',  ( 46.00000000000000711, 20.00000000000000000, 51.00000000000000000 ) ) ;
#45849=DIRECTION ( 'NONE',  ( -0.000000000000000000, 1.000000000000000000, -0.000000000000000000 ) ) ;
#45964=VECTOR ( 'NONE', #40269, 1000.000000000000000 ) ;
#45985=FACE_OUTER_BOUND ( 'NONE', #34525, .T. ) ;
#46037=( NAMED_UNIT ( * ) SI_UNIT ( $, .STERADIAN. ) SOLID_ANGLE_UNIT ( ) );
#46052=CARTESIAN_POINT ( 'NONE',  ( -46.00000000000000711, 0.000000000000000000, -4.999999999999988454 ) ) ;
#46068=CARTESIAN_POINT ( 'NONE',  ( 1.734723475976807489E-15, -43.50000000000000000, -30.00000000000000711 ) ) ;
#46109=ORIENTED_EDGE ( 'NONE', *, *, #37169, .T. ) ;
#46136=AXIS2_PLACEMENT_3D ( 'NONE', #46068, #28767, #49026 ) ;
#46177=EDGE_LOOP ( 'NONE', ( #11667, #32399 ) ) ;
#46232=DIRECTION ( 'NONE',  ( -0.000000000000000000, -1.000000000000000000, -0.000000000000000000 ) ) ;
#46276=DIRECTION ( 'NONE',  ( -0.000000000000000000, -1.000000000000000000, -0.000000000000000000 ) ) ;
#46324=ORIENTED_EDGE ( 'NONE', *, *, #9124, .T. ) ;
#46348=VECTOR ( 'NONE', #36773, 1000.000000000000000 ) ;
#46452=DIRECTION ( 'NONE',  ( 0.000000000000000000, 0.000000000000000000, 1.000000000000000000 ) ) ;
#46486=APPLICATION_CONTEXT ( 'automotive_design' ) ;
#46498=DIRECTION ( 'NONE',  ( 0.000000000000000000, 0.000000000000000000, 1.000000000000000000 ) ) ;
#46542=VECTOR ( 'NONE', #10565, 1000.000000000000000 ) ;
#46568=DIRECTION ( 'NONE',  ( 0.000000000000000000, 0.000000000000000000, -1.000000000000000000 ) ) ;
#46644=CARTESIAN_POINT ( 'NONE',  ( -30.00000000000000000, -43.50000000000000000, 0.000000000000000000 ) ) ;
#46647=DIRECTION ( 'NONE',  ( 0.000000000000000000, 1.000000000000000000, 0.000000000000000000 ) ) ;
#46903=ORIENTED_EDGE ( 'NONE', *, *, #17172, .T. ) ;
#46908=DIRECTION ( 'NONE',  ( 1.000000000000000000, -0.000000000000000000, 0.000000000000000000 ) ) ;
#46912=PRODUCT_DEFINITION_CONTEXT ( 'detailed design', #46486, 'design' ) ;
#46971=EDGE_CURVE ( 'NONE', #31192, #28668, #42359, .T. ) ;
#46991=ORIENTED_EDGE ( 'NONE', *, *, #31993, .T. ) ;
#47167=VERTEX_POINT ( 'NONE', #5818 ) ;
#47208=CARTESIAN_POINT ( 'NONE',  ( 0.000000000000000000, 20.00000000000000000, 0.000000000000000000 ) ) ;
#47242=ORIENTED_EDGE ( 'NONE', *, *, #49043, .F. ) ;
#47263=AXIS2_PLACEMENT_3D ( 'NONE', #35652, #35390, #43285 ) ;
#47281=AXIS2_PLACEMENT_3D ( 'NONE', #14235, #41550, #13707 ) ;
#47326=CARTESIAN_POINT ( 'NONE',  ( 46.00000000000000711, 20.00000000000000000, 46.00000000000000000 ) ) ;
#47356=ORIENTED_EDGE ( 'NONE', *, *, #23553, .T. ) ;
#47412=DIRECTION ( 'NONE',  ( 1.000000000000000000, -0.000000000000000000, 0.000000000000000000 ) ) ;
#47435=CARTESIAN_POINT ( 'NONE',  ( 46.00000000000000711, 20.00000000000000000, -46.00000000000000000 ) ) ;
#47442=ORIENTED_EDGE ( 'NONE', *, *, #8551, .T. ) ;
#47466=CARTESIAN_POINT ( 'NONE',  ( -46.00000000000000711, 20.00000000000000000, 8.673617379884035472E-15 ) ) ;
#47487=CARTESIAN_POINT ( 'NONE',  ( 1.734723475976807094E-15, 20.00000000000000000, 41.00000000000000711 ) ) ;
#47620=EDGE_CURVE ( 'NONE', #21250, #1126, #11322, .T. ) ;
#47655=DIRECTION ( 'NONE',  ( 0.000000000000000000, 1.000000000000000000, 0.000000000000000000 ) ) ;
#47762=VECTOR ( 'NONE', #33587, 1000.000000000000000 ) ;
#47805=CARTESIAN_POINT ( 'NONE',  ( 46.00000000000000711, 0.000000000000000000, 51.00000000000000000 ) ) ;
#47809=VECTOR ( 'NONE', #18315, 1000.000000000000000 ) ;
#47828=CARTESIAN_POINT ( 'NONE',  ( 2.449293598294706119E-15, 20.00000000000000355, -20.00000000000000000 ) ) ;
#47891=CARTESIAN_POINT ( 'NONE',  ( 60.00000000000001421, -63.50000000000000000, 60.00000000000000711 ) ) ;
#47895=LINE ( 'NONE', #11100, #48727 ) ;
#47931=CARTESIAN_POINT ( 'NONE',  ( 0.000000000000000000, -63.50000000000000000, -60.00000000000000711 ) ) ;
#48038=ORIENTED_EDGE ( 'NONE', *, *, #10832, .F. ) ;
#48130=LINE ( 'NONE', #3985, #9712 ) ;
#48201=EDGE_LOOP ( 'NONE', ( #44563, #50376, #16254, #36007 ) ) ;
#48217=DIRECTION ( 'NONE',  ( 0.000000000000000000, 0.000000000000000000, -1.000000000000000000 ) ) ;
#48358=CARTESIAN_POINT ( 'NONE',  ( -46.00000000000000711, 20.00000000000000000, 8.673617379884035472E-15 ) ) ;
#48599=ORIENTED_EDGE ( 'NONE', *, *, #30163, .T. ) ;
#48600=FACE_OUTER_BOUND ( 'NONE', #36889, .T. ) ;
#48607=VECTOR ( 'NONE', #24689, 1000.000000000000000 ) ;
#48612=CARTESIAN_POINT ( 'NONE',  ( 30.00000000000000711, -43.50000000000000000, 30.00000000000000355 ) ) ;
#48676=CARTESIAN_POINT ( 'NONE',  ( 46.00000000000000711, 20.00000000000000000, -51.00000000000000000 ) ) ;
#48681=CARTESIAN_POINT ( 'NONE',  ( 3.686287386450715076E-15, 0.000000000000000000, -46.00000000000000711 ) ) ;
#48702=VERTEX_POINT ( 'NONE', #44398 ) ;
#48724=LINE ( 'NONE', #51626, #30919 ) ;
#48727=VECTOR ( 'NONE', #15078, 1000.000000000000000 ) ;
#48737=CARTESIAN_POINT ( 'NONE',  ( 60.00000000000001421, -63.50000000000000000, 0.000000000000000000 ) ) ;
#48759=DIRECTION ( 'NONE',  ( 0.000000000000000000, 1.000000000000000000, -0.000000000000000000 ) ) ;
#48801=FACE_OUTER_BOUND ( 'NONE', #44634, .T. ) ;
#48814=ORIENTED_EDGE ( 'NONE', *, *, #27494, .T. ) ;
#48846=DIRECTION ( 'NONE',  ( 0.000000000000000000, 0.000000000000000000, 1.000000000000000000 ) ) ;
#48856=DIRECTION ( 'NONE',  ( 0.000000000000000000, 0.000000000000000000, -1.000000000000000000 ) ) ;
#48869=EDGE_CURVE ( 'NONE', #2101, #10970, #31471, .T. ) ;
#48902=CARTESIAN_POINT ( 'NONE',  ( -60.00000000000000000, -63.50000000000000000, -60.00000000000000711 ) ) ;
#48934=DIRECTION ( 'NONE',  ( -1.000000000000000000, -0.000000000000000000, -0.000000000000000000 ) ) ;
#48953=PLANE ( 'NONE',  #31172 ) ;
#48995=LINE ( 'NONE', #45065, #23862 ) ;
#49026=DIRECTION ( 'NONE',  ( 1.000000000000000000, 0.000000000000000000, 5.782411586589357392E-17 ) ) ;
#49043=EDGE_CURVE ( 'NONE', #18767, #24959, #19376, .T. ) ;
#49107=ORIENTED_EDGE ( 'NONE', *, *, #45270, .F. ) ;
#49154=ORIENTED_EDGE ( 'NONE', *, *, #25952, .F. ) ;
#49169=CARTESIAN_POINT ( 'NONE',  ( 46.00000000000000711, 20.00000000000000000, -41.00000000000000000 ) ) ;
#49287=ORIENTED_EDGE ( 'NONE', *, *, #36192, .T. ) ;
#49327=DIRECTION ( 'NONE',  ( -0.000000000000000000, -1.000000000000000000, -0.000000000000000000 ) ) ;
#49363=CARTESIAN_POINT ( 'NONE',  ( -60.00000000000000000, -43.50000000000000000, -60.00000000000000711 ) ) ;
#49477=AXIS2_PLACEMENT_3D ( 'NONE', #6553, #43308, #39604 ) ;
#49490=ADVANCED_FACE ( 'NONE', ( #41027 ), #1080, .F. ) ;
#49524=PLANE ( 'NONE',  #22830 ) ;
#49527=DIRECTION ( 'NONE',  ( 1.000000000000000000, -0.000000000000000000, 0.000000000000000000 ) ) ;
#49556=ORIENTED_EDGE ( 'NONE', *, *, #32735, .T. ) ;
#49652=PLANE ( 'NONE',  #15195 ) ;
#49666=CARTESIAN_POINT ( 'NONE',  ( -46.00000000000000711, 20.00000000000000000, -4.999999999999988454 ) ) ;
#49672=CIRCLE ( 'NONE', #11911, 20.00000000000000000 ) ;
#49679=VECTOR ( 'NONE', #24914, 1000.000000000000000 ) ;
#49732=DIRECTION ( 'NONE',  ( -0.000000000000000000, 1.000000000000000000, -0.000000000000000000 ) ) ;
#49760=CARTESIAN_POINT ( 'NONE',  ( -30.00000000000000000, -43.50000000000000000, -30.00000000000000711 ) ) ;
#49796=FACE_OUTER_BOUND ( 'NONE', #4931, .T. ) ;
#49851=AXIS2_PLACEMENT_3D ( 'NONE', #30609, #23003, #30113 ) ;
#49902=ORIENTED_EDGE ( 'NONE', *, *, #1921, .T. ) ;
#49905=FACE_BOUND ( 'NONE', #17052, .T. ) ;
#49942=ORIENTED_EDGE ( 'NONE', *, *, #23614, .F. ) ;
#49951=AXIS2_PLACEMENT_3D ( 'NONE', #5761, #6529, #10445 ) ;
#49956=FILL_AREA_STYLE ('',( #41274 ) ) ;
#49968=DIRECTION ( 'NONE',  ( 0.000000000000000000, 1.000000000000000000, 0.000000000000000000 ) ) ;
#49999=PLANE ( 'NONE',  #46136 ) ;
#50015=VECTOR ( 'NONE', #27689, 1000.000000000000000 ) ;
#50027=ORIENTED_EDGE ( 'NONE', *, *, #19576, .F. ) ;
#50055=ORIENTED_EDGE ( 'NONE', *, *, #38474, .F. ) ;
#50069=CYLINDRICAL_SURFACE ( 'NONE', #5901, 4.999999999999997335 ) ;
#50196=DIRECTION ( 'NONE',  ( 0.000000000000000000, 0.000000000000000000, -1.000000000000000000 ) ) ;
#50294=DIRECTION ( 'NONE',  ( 0.000000000000000000, 1.000000000000000000, 0.000000000000000000 ) ) ;
#50330=VECTOR ( 'NONE', #27985, 1000.000000000000000 ) ;
#50376=ORIENTED_EDGE ( 'NONE', *, *, #6854, .F. ) ;
#50405=ADVANCED_FACE ( 'NONE', ( #20946 ), #36966, .F. ) ;
#50558=CARTESIAN_POINT ( 'NONE',  ( 0.000000000000000000, -43.50000000000000000, 30.00000000000000355 ) ) ;
#50654=ORIENTED_EDGE ( 'NONE', *, *, #3409, .F. ) ;
#50691=DIRECTION ( 'NONE',  ( 0.000000000000000000, 0.000000000000000000, -1.000000000000000000 ) ) ;
#50707=CARTESIAN_POINT ( 'NONE',  ( 60.00000000000001421, 20.00000000000000000, 60.00000000000000711 ) ) ;
#50751=AXIS2_PLACEMENT_3D ( 'NONE', #48737, #49527, #16935 ) ;
#50842=DIRECTION ( 'NONE',  ( 0.000000000000000000, 0.000000000000000000, -1.000000000000000000 ) ) ;
#50877=AXIS2_PLACEMENT_3D ( 'NONE', #3541, #19827, #22746 ) ;
#50882=ORIENTED_EDGE ( 'NONE', *, *, #40003, .T. ) ;
#50891=DIRECTION ( 'NONE',  ( 0.000000000000000000, -0.000000000000000000, -1.000000000000000000 ) ) ;
#50951=AXIS2_PLACEMENT_3D ( 'NONE', #27380, #43432, #15310 ) ;
#50968=AXIS2_PLACEMENT_3D ( 'NONE', #11729, #16738, #3855 ) ;
#50996=LINE ( 'NONE', #6066, #38753 ) ;
#51023=VERTEX_POINT ( 'NONE', #49169 ) ;
#51027=AXIS2_PLACEMENT_3D ( 'NONE', #38205, #2214, #19026 ) ;
#51085=CARTESIAN_POINT ( 'NONE',  ( -60.00000000000000000, 0.000000000000000000, -60.00000000000000711 ) ) ;
#51107=VERTEX_POINT ( 'NONE', #11209 ) ;
#51228=EDGE_CURVE ( 'NONE', #28668, #40958, #14051, .T. ) ;
#51314=ADVANCED_FACE ( 'NONE', ( #690 ), #36162, .F. ) ;
#51385=ORIENTED_EDGE ( 'NONE', *, *, #43648, .T. ) ;
#51405=AXIS2_PLACEMENT_3D ( 'NONE', #39928, #511, #16572 ) ;
#51608=PLANE ( 'NONE',  #10243 ) ;
#51626=CARTESIAN_POINT ( 'NONE',  ( 60.00000000000001421, 20.00000000000000000, 60.00000000000000711 ) ) ;
#51630=VECTOR ( 'NONE', #27246, 1000.000000000000000 ) ;
#51728=CIRCLE ( 'NONE', #44172, 20.00000000000000000 ) ;
#51787=VERTEX_POINT ( 'NONE', #49760 ) ;
#51816=ORIENTED_EDGE ( 'NONE', *, *, #37609, .T. ) ;
#51930=CARTESIAN_POINT ( 'NONE',  ( 46.00000000000000000, 20.00000000000000000, 4.999999999999997335 ) ) ;
#51938=DIRECTION ( 'NONE',  ( -0.000000000000000000, 0.000000000000000000, 1.000000000000000000 ) ) ;
#51946=CARTESIAN_POINT ( 'NONE',  ( 4.298610786024391605E-15, 0.000000000000000000, -41.00000000000000711 ) ) ;
ENDSEC;
END-ISO-10303-21;
